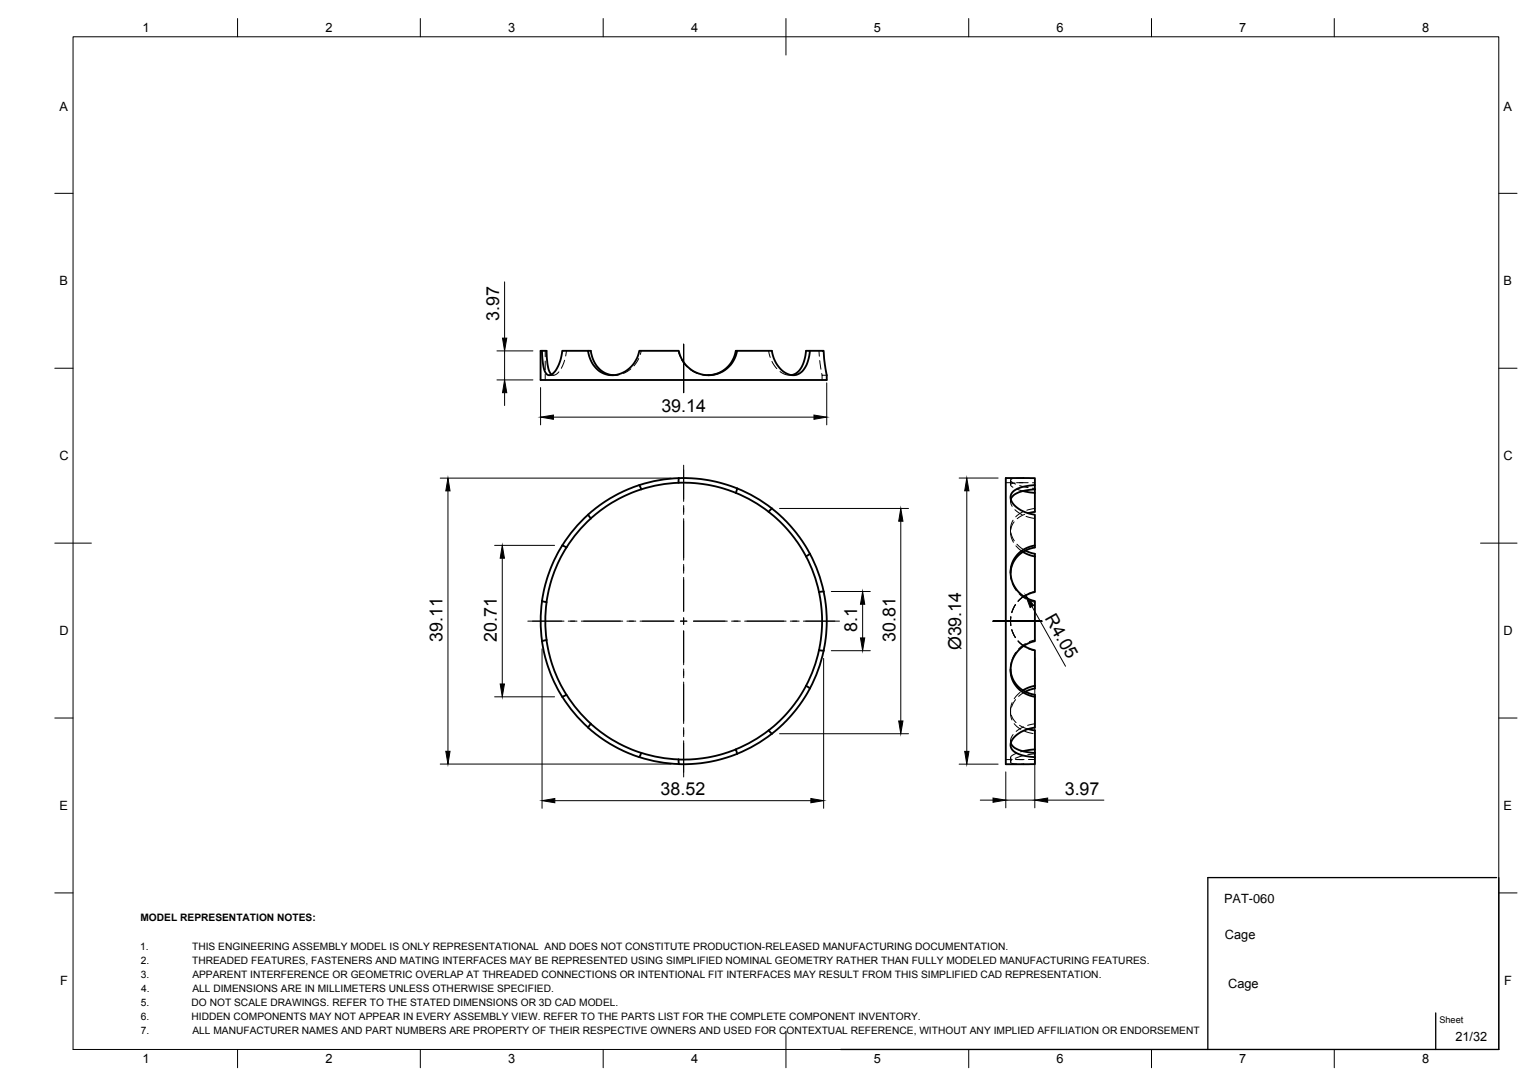
ISO-10303-21;
HEADER;
/* Generated by software containing ST-Developer
 * from STEP Tools, Inc. (www.steptools.com) 
 */

FILE_DESCRIPTION(
/* description */ ('Indexing fixture plate with plunger'),
/* implementation_level */ '2;1');

FILE_NAME(
/* name */ 'Cage.step',
/* time_stamp */ '2026-10-28T03:23:41-07:00',
/* author */ (''),
/* organization */ (''),
/* preprocessor_version */ 'ST-DEVELOPER v20.2',
/* originating_system */ 'Autodesk Translation Framework v15.17.0.0',
/* authorisation */ '');

FILE_SCHEMA (('AUTOMOTIVE_DESIGN { 1 0 10303 214 3 1 1 }'));
ENDSEC;

DATA;
#10=MECHANICAL_DESIGN_GEOMETRIC_PRESENTATION_REPRESENTATION('',(#341),#10020);
#204=SPHERICAL_SURFACE('',#5145,0.412776);
#205=SPHERICAL_SURFACE('',#5163,0.412776);
#206=SPHERICAL_SURFACE('',#5168,0.412776);
#207=SPHERICAL_SURFACE('',#5173,0.412776);
#208=SPHERICAL_SURFACE('',#5179,0.412776);
#209=SPHERICAL_SURFACE('',#5184,0.412776);
#210=SPHERICAL_SURFACE('',#5189,0.412776);
#211=SPHERICAL_SURFACE('',#5194,0.412776);
#212=SPHERICAL_SURFACE('',#5202,0.412776);
#240=B_SPLINE_CURVE_WITH_KNOTS('',3,(#8709,#8710,#8711,#8712,#8713,#8714,
#8715,#8716,#8717,#8718,#8719,#8720,#8721,#8722,#8723,#8724,#8725,#8726,
#8727,#8728,#8729,#8730),.UNSPECIFIED.,.F.,.F.,(4,2,2,2,2,2,2,2,2,2,4),
(0.0789043916784349,0.21052649634152,0.31578974451228,0.421052992683041,
0.522171766675512,0.623290540667983,0.724409314660453,0.825528088652924,
0.930791336823684,1.03605458499444,1.16767668965753),.UNSPECIFIED.);
#241=B_SPLINE_CURVE_WITH_KNOTS('',3,(#8734,#8735,#8736,#8737,#8738,#8739,
#8740,#8741,#8742,#8743,#8744,#8745,#8746,#8747,#8748,#8749,#8750,#8751,
#8752,#8753,#8754,#8755),.UNSPECIFIED.,.F.,.F.,(4,2,2,2,2,2,2,2,2,2,4),
(0.0774711646211702,0.142095081356994,0.284190162713987,0.410912155766437,
0.514012992401139,0.617113829035841,0.720214665670543,0.823315502305246,
0.950037495357694,1.09213257671469,1.15675649345051),.UNSPECIFIED.);
#242=B_SPLINE_CURVE_WITH_KNOTS('',3,(#8761,#8762,#8763,#8764,#8765,#8766,
#8767,#8768,#8769,#8770,#8771,#8772,#8773,#8774,#8775,#8776,#8777,#8778,
#8779,#8780,#8781,#8782),.UNSPECIFIED.,.F.,.F.,(4,2,2,2,2,2,2,2,2,2,4),
(0.0774711646211703,0.142095081356994,0.284190162713988,0.410912155766436,
0.514012992401139,0.617113829035841,0.720214665670544,0.823315502305246,
0.950037495357695,1.09213257671469,1.15675649345051),.UNSPECIFIED.);
#243=B_SPLINE_CURVE_WITH_KNOTS('',3,(#8786,#8787,#8788,#8789,#8790,#8791,
#8792,#8793,#8794,#8795,#8796,#8797,#8798,#8799,#8800,#8801,#8802,#8803,
#8804,#8805,#8806,#8807),.UNSPECIFIED.,.F.,.F.,(4,2,2,2,2,2,2,2,2,2,4),
(0.0774711646211702,0.142095081356994,0.284190162713988,0.410912155766436,
0.514012992401139,0.617113829035841,0.720214665670544,0.823315502305246,
0.950037495357695,1.09213257671469,1.15675649345051),.UNSPECIFIED.);
#244=B_SPLINE_CURVE_WITH_KNOTS('',3,(#8811,#8812,#8813,#8814,#8815,#8816,
#8817,#8818,#8819,#8820,#8821,#8822,#8823,#8824,#8825,#8826,#8827,#8828,
#8829,#8830,#8831,#8832),.UNSPECIFIED.,.F.,.F.,(4,2,2,2,2,2,2,2,2,2,4),
(0.0774711646211702,0.142095081356994,0.284190162713988,0.410912155766436,
0.514012992401139,0.617113829035842,0.720214665670544,0.823315502305246,
0.950037495357696,1.09213257671469,1.15675649345051),.UNSPECIFIED.);
#245=B_SPLINE_CURVE_WITH_KNOTS('',3,(#8841,#8842,#8843,#8844,#8845,#8846,
#8847,#8848,#8849,#8850,#8851,#8852,#8853,#8854,#8855,#8856,#8857,#8858,
#8859,#8860,#8861,#8862),.UNSPECIFIED.,.F.,.F.,(4,2,2,2,2,2,2,2,2,2,4),
(0.0774711646211702,0.142095081356994,0.284190162713987,0.410912155766436,
0.514012992401139,0.617113829035841,0.720214665670543,0.823315502305246,
0.950037495357695,1.09213257671469,1.15675649345051),.UNSPECIFIED.);
#246=B_SPLINE_CURVE_WITH_KNOTS('',3,(#8866,#8867,#8868,#8869,#8870,#8871,
#8872,#8873,#8874,#8875,#8876,#8877,#8878,#8879,#8880,#8881,#8882,#8883,
#8884,#8885,#8886,#8887),.UNSPECIFIED.,.F.,.F.,(4,2,2,2,2,2,2,2,2,2,4),
(0.0774711646211702,0.142095081356994,0.284190162713987,0.410912155766436,
0.514012992401139,0.617113829035841,0.720214665670543,0.823315502305246,
0.950037495357695,1.09213257671469,1.15675649345051),.UNSPECIFIED.);
#247=B_SPLINE_CURVE_WITH_KNOTS('',3,(#8891,#8892,#8893,#8894,#8895,#8896,
#8897,#8898,#8899,#8900,#8901,#8902,#8903,#8904,#8905,#8906,#8907,#8908,
#8909,#8910,#8911,#8912),.UNSPECIFIED.,.F.,.F.,(4,2,2,2,2,2,2,2,2,2,4),
(0.0774711646211703,0.142095081356994,0.284190162713988,0.410912155766437,
0.514012992401139,0.617113829035841,0.720214665670544,0.823315502305247,
0.950037495357696,1.09213257671469,1.15675649345051),.UNSPECIFIED.);
#248=B_SPLINE_CURVE_WITH_KNOTS('',3,(#8916,#8917,#8918,#8919,#8920,#8921,
#8922,#8923,#8924,#8925,#8926,#8927,#8928,#8929,#8930,#8931,#8932,#8933,
#8934,#8935,#8936,#8937),.UNSPECIFIED.,.F.,.F.,(4,2,2,2,2,2,2,2,2,2,4),
(0.0774711646211703,0.142095081356994,0.284190162713987,0.410912155766436,
0.514012992401139,0.617113829035841,0.720214665670543,0.823315502305245,
0.950037495357694,1.09213257671469,1.15675649345051),.UNSPECIFIED.);
#249=B_SPLINE_CURVE_WITH_KNOTS('',3,(#8941,#8942,#8943,#8944,#8945,#8946,
#8947,#8948,#8949,#8950,#8951,#8952,#8953,#8954,#8955,#8956,#8957,#8958,
#8959,#8960,#8961,#8962),.UNSPECIFIED.,.F.,.F.,(4,2,2,2,2,2,2,2,2,2,4),
(0.0774711646211703,0.142095081356994,0.284190162713988,0.410912155766437,
0.514012992401139,0.617113829035841,0.720214665670544,0.823315502305246,
0.950037495357695,1.09213257671469,1.15675649345051),.UNSPECIFIED.);
#250=B_SPLINE_CURVE_WITH_KNOTS('',3,(#8970,#8971,#8972,#8973,#8974,#8975,
#8976,#8977,#8978,#8979,#8980,#8981,#8982,#8983,#8984,#8985,#8986,#8987,
#8988,#8989,#8990,#8991),.UNSPECIFIED.,.F.,.F.,(4,2,2,2,2,2,2,2,2,2,4),
(0.0789043916784349,0.21052649634152,0.315789744512281,0.421052992683041,
0.522171766675512,0.623290540667983,0.724409314660453,0.825528088652924,
0.930791336823684,1.03605458499444,1.16767668965753),.UNSPECIFIED.);
#251=B_SPLINE_CURVE_WITH_KNOTS('',3,(#8999,#9000,#9001,#9002,#9003,#9004,
#9005,#9006,#9007,#9008,#9009,#9010,#9011,#9012,#9013,#9014,#9015,#9016,
#9017,#9018,#9019,#9020),.UNSPECIFIED.,.F.,.F.,(4,2,2,2,2,2,2,2,2,2,4),
(0.0789043916784348,0.210526496341521,0.315789744512281,0.421052992683042,
0.522171766675513,0.623290540667983,0.724409314660454,0.825528088652925,
0.930791336823685,1.03605458499444,1.16767668965753),.UNSPECIFIED.);
#252=B_SPLINE_CURVE_WITH_KNOTS('',3,(#9028,#9029,#9030,#9031,#9032,#9033,
#9034,#9035,#9036,#9037,#9038,#9039,#9040,#9041,#9042,#9043,#9044,#9045,
#9046,#9047,#9048,#9049),.UNSPECIFIED.,.F.,.F.,(4,2,2,2,2,2,2,2,2,2,4),
(0.0789043916784349,0.21052649634152,0.31578974451228,0.421052992683041,
0.522171766675511,0.623290540667982,0.724409314660453,0.825528088652924,
0.930791336823685,1.03605458499444,1.16767668965753),.UNSPECIFIED.);
#253=B_SPLINE_CURVE_WITH_KNOTS('',3,(#9059,#9060,#9061,#9062,#9063,#9064,
#9065,#9066,#9067,#9068,#9069,#9070,#9071,#9072,#9073,#9074,#9075,#9076,
#9077,#9078,#9079,#9080),.UNSPECIFIED.,.F.,.F.,(4,2,2,2,2,2,2,2,2,2,4),
(0.0789043916784348,0.21052649634152,0.315789744512281,0.421052992683041,
0.522171766675511,0.623290540667982,0.724409314660453,0.825528088652924,
0.930791336823684,1.03605458499444,1.16767668965753),.UNSPECIFIED.);
#254=B_SPLINE_CURVE_WITH_KNOTS('',3,(#9088,#9089,#9090,#9091,#9092,#9093,
#9094,#9095,#9096,#9097,#9098,#9099,#9100,#9101,#9102,#9103,#9104,#9105,
#9106,#9107,#9108,#9109),.UNSPECIFIED.,.F.,.F.,(4,2,2,2,2,2,2,2,2,2,4),
(0.0789043916784348,0.21052649634152,0.31578974451228,0.42105299268304,
0.522171766675511,0.623290540667982,0.724409314660453,0.825528088652924,
0.930791336823684,1.03605458499444,1.16767668965753),.UNSPECIFIED.);
#255=B_SPLINE_CURVE_WITH_KNOTS('',3,(#9117,#9118,#9119,#9120,#9121,#9122,
#9123,#9124,#9125,#9126,#9127,#9128,#9129,#9130,#9131,#9132,#9133,#9134,
#9135,#9136,#9137,#9138),.UNSPECIFIED.,.F.,.F.,(4,2,2,2,2,2,2,2,2,2,4),
(0.0789043916784348,0.21052649634152,0.315789744512281,0.421052992683041,
0.522171766675512,0.623290540667982,0.724409314660453,0.825528088652924,
0.930791336823684,1.03605458499444,1.16767668965753),.UNSPECIFIED.);
#256=B_SPLINE_CURVE_WITH_KNOTS('',3,(#9146,#9147,#9148,#9149,#9150,#9151,
#9152,#9153,#9154,#9155,#9156,#9157,#9158,#9159,#9160,#9161,#9162,#9163,
#9164,#9165,#9166,#9167),.UNSPECIFIED.,.F.,.F.,(4,2,2,2,2,2,2,2,2,2,4),
(0.0789043916784349,0.21052649634152,0.31578974451228,0.42105299268304,
0.522171766675511,0.623290540667982,0.724409314660453,0.825528088652924,
0.930791336823684,1.03605458499444,1.16767668965753),.UNSPECIFIED.);
#257=B_SPLINE_CURVE_WITH_KNOTS('',3,(#9176,#9177,#9178,#9179,#9180,#9181,
#9182,#9183,#9184,#9185,#9186,#9187,#9188,#9189,#9190,#9191,#9192,#9193,
#9194,#9195,#9196,#9197),.UNSPECIFIED.,.F.,.F.,(4,2,2,2,2,2,2,2,2,2,4),
(0.0789043916784348,0.21052649634152,0.31578974451228,0.42105299268304,
0.522171766675511,0.623290540667982,0.724409314660453,0.825528088652924,
0.930791336823684,1.03605458499444,1.16767668965753),.UNSPECIFIED.);
#279=SHAPE_REPRESENTATION_RELATIONSHIP('SRR','None',#10154,#306);
#306=ADVANCED_BREP_SHAPE_REPRESENTATION('',(#376),#10007);
#341=STYLED_ITEM('',(#10368),#376);
#376=MANIFOLD_SOLID_BREP('Continuous crown cage',#4596);
#435=FACE_BOUND('',#1135,.T.);
#587=PLANE('',#5160);
#588=PLANE('',#5165);
#589=PLANE('',#5170);
#590=PLANE('',#5175);
#591=PLANE('',#5181);
#592=PLANE('',#5186);
#593=PLANE('',#5191);
#594=PLANE('',#5200);
#595=PLANE('',#5204);
#596=PLANE('',#5205);
#781=FACE_OUTER_BOUND('',#1115,.T.);
#782=FACE_OUTER_BOUND('',#1116,.T.);
#783=FACE_OUTER_BOUND('',#1117,.T.);
#784=FACE_OUTER_BOUND('',#1118,.T.);
#785=FACE_OUTER_BOUND('',#1119,.T.);
#786=FACE_OUTER_BOUND('',#1120,.T.);
#787=FACE_OUTER_BOUND('',#1121,.T.);
#788=FACE_OUTER_BOUND('',#1122,.T.);
#789=FACE_OUTER_BOUND('',#1123,.T.);
#790=FACE_OUTER_BOUND('',#1124,.T.);
#791=FACE_OUTER_BOUND('',#1125,.T.);
#792=FACE_OUTER_BOUND('',#1126,.T.);
#793=FACE_OUTER_BOUND('',#1127,.T.);
#794=FACE_OUTER_BOUND('',#1128,.T.);
#795=FACE_OUTER_BOUND('',#1129,.T.);
#796=FACE_OUTER_BOUND('',#1130,.T.);
#797=FACE_OUTER_BOUND('',#1131,.T.);
#798=FACE_OUTER_BOUND('',#1132,.T.);
#799=FACE_OUTER_BOUND('',#1133,.T.);
#800=FACE_OUTER_BOUND('',#1134,.T.);
#801=FACE_OUTER_BOUND('',#1136,.T.);
#1115=EDGE_LOOP('',(#3453,#3454,#3455,#3456));
#1116=EDGE_LOOP('',(#3457,#3458,#3459,#3460,#3461,#3462,#3463,#3464,#3465,
#3466,#3467,#3468,#3469,#3470,#3471,#3472,#3473,#3474,#3475,#3476,#3477,
#3478));
#1117=EDGE_LOOP('',(#3479,#3480,#3481,#3482));
#1118=EDGE_LOOP('',(#3483,#3484,#3485,#3486));
#1119=EDGE_LOOP('',(#3487,#3488,#3489,#3490));
#1120=EDGE_LOOP('',(#3491,#3492,#3493,#3494));
#1121=EDGE_LOOP('',(#3495,#3496,#3497,#3498));
#1122=EDGE_LOOP('',(#3499,#3500,#3501,#3502));
#1123=EDGE_LOOP('',(#3503,#3504,#3505,#3506,#3507,#3508));
#1124=EDGE_LOOP('',(#3509,#3510,#3511,#3512));
#1125=EDGE_LOOP('',(#3513,#3514,#3515,#3516));
#1126=EDGE_LOOP('',(#3517,#3518,#3519,#3520));
#1127=EDGE_LOOP('',(#3521,#3522,#3523,#3524));
#1128=EDGE_LOOP('',(#3525,#3526,#3527,#3528));
#1129=EDGE_LOOP('',(#3529,#3530,#3531,#3532));
#1130=EDGE_LOOP('',(#3533,#3534,#3535,#3536));
#1131=EDGE_LOOP('',(#3537,#3538,#3539,#3540,#3541,#3542,#3543,#3544,#3545,
#3546,#3547,#3548,#3549,#3550,#3551,#3552,#3553,#3554,#3555,#3556,#3557,
#3558));
#1132=EDGE_LOOP('',(#3559,#3560,#3561,#3562));
#1133=EDGE_LOOP('',(#3563,#3564,#3565,#3566));
#1134=EDGE_LOOP('',(#3567));
#1135=EDGE_LOOP('',(#3568));
#1136=EDGE_LOOP('',(#3569,#3570,#3571,#3572));
#1473=LINE('',#8836,#1693);
#1474=LINE('',#9172,#1694);
#1693=VECTOR('',#6146,1.956752);
#1694=VECTOR('',#6237,1.893248);
#1940=CIRCLE('',#5146,0.405071403305639);
#1941=CIRCLE('',#5147,0.405071403305639);
#1942=CIRCLE('',#5149,1.956752);
#1943=CIRCLE('',#5150,1.956752);
#1944=CIRCLE('',#5151,1.956752);
#1945=CIRCLE('',#5152,1.956752);
#1946=CIRCLE('',#5153,1.956752);
#1947=CIRCLE('',#5154,1.956752);
#1948=CIRCLE('',#5155,1.956752);
#1949=CIRCLE('',#5156,1.956752);
#1950=CIRCLE('',#5157,1.956752);
#1951=CIRCLE('',#5158,1.956752);
#1952=CIRCLE('',#5159,1.956752);
#1953=CIRCLE('',#5161,1.893248);
#1954=CIRCLE('',#5162,0.405071403305639);
#1955=CIRCLE('',#5164,0.405071403305639);
#1956=CIRCLE('',#5166,1.893248);
#1957=CIRCLE('',#5167,0.405071403305639);
#1958=CIRCLE('',#5169,0.405071403305639);
#1959=CIRCLE('',#5171,1.893248);
#1960=CIRCLE('',#5172,0.405071403305639);
#1961=CIRCLE('',#5174,0.405071403305639);
#1962=CIRCLE('',#5176,1.893248);
#1963=CIRCLE('',#5177,1.893248);
#1964=CIRCLE('',#5178,0.405071403305639);
#1965=CIRCLE('',#5180,0.405071403305639);
#1966=CIRCLE('',#5182,1.893248);
#1967=CIRCLE('',#5183,0.405071403305639);
#1968=CIRCLE('',#5185,0.405071403305639);
#1969=CIRCLE('',#5187,1.893248);
#1970=CIRCLE('',#5188,0.405071403305639);
#1971=CIRCLE('',#5190,0.405071403305639);
#1972=CIRCLE('',#5192,1.893248);
#1973=CIRCLE('',#5193,0.405071403305639);
#1974=CIRCLE('',#5195,0.405071403305639);
#1975=CIRCLE('',#5197,1.893248);
#1976=CIRCLE('',#5198,1.893248);
#1977=CIRCLE('',#5199,1.893248);
#1978=CIRCLE('',#5201,0.405071403305639);
#1979=CIRCLE('',#5203,0.405071403305639);
#2275=VERTEX_POINT('',#8707);
#2276=VERTEX_POINT('',#8708);
#2277=VERTEX_POINT('',#8731);
#2278=VERTEX_POINT('',#8733);
#2279=VERTEX_POINT('',#8758);
#2280=VERTEX_POINT('',#8760);
#2281=VERTEX_POINT('',#8783);
#2282=VERTEX_POINT('',#8785);
#2283=VERTEX_POINT('',#8808);
#2284=VERTEX_POINT('',#8810);
#2285=VERTEX_POINT('',#8833);
#2286=VERTEX_POINT('',#8835);
#2287=VERTEX_POINT('',#8838);
#2288=VERTEX_POINT('',#8840);
#2289=VERTEX_POINT('',#8863);
#2290=VERTEX_POINT('',#8865);
#2291=VERTEX_POINT('',#8888);
#2292=VERTEX_POINT('',#8890);
#2293=VERTEX_POINT('',#8913);
#2294=VERTEX_POINT('',#8915);
#2295=VERTEX_POINT('',#8938);
#2296=VERTEX_POINT('',#8940);
#2297=VERTEX_POINT('',#8965);
#2298=VERTEX_POINT('',#8969);
#2299=VERTEX_POINT('',#8994);
#2300=VERTEX_POINT('',#8998);
#2301=VERTEX_POINT('',#9023);
#2302=VERTEX_POINT('',#9027);
#2303=VERTEX_POINT('',#9052);
#2304=VERTEX_POINT('',#9054);
#2305=VERTEX_POINT('',#9058);
#2306=VERTEX_POINT('',#9083);
#2307=VERTEX_POINT('',#9087);
#2308=VERTEX_POINT('',#9112);
#2309=VERTEX_POINT('',#9116);
#2310=VERTEX_POINT('',#9141);
#2311=VERTEX_POINT('',#9145);
#2312=VERTEX_POINT('',#9170);
#2313=VERTEX_POINT('',#9173);
#2314=VERTEX_POINT('',#9175);
#2706=EDGE_CURVE('',#2275,#2276,#240,.T.);
#2707=EDGE_CURVE('',#2277,#2275,#1940,.T.);
#2708=EDGE_CURVE('',#2278,#2277,#241,.T.);
#2709=EDGE_CURVE('',#2276,#2278,#1941,.T.);
#2710=EDGE_CURVE('',#2279,#2277,#1942,.T.);
#2711=EDGE_CURVE('',#2279,#2280,#242,.T.);
#2712=EDGE_CURVE('',#2281,#2280,#1943,.T.);
#2713=EDGE_CURVE('',#2281,#2282,#243,.T.);
#2714=EDGE_CURVE('',#2283,#2282,#1944,.T.);
#2715=EDGE_CURVE('',#2283,#2284,#244,.T.);
#2716=EDGE_CURVE('',#2285,#2284,#1945,.T.);
#2717=EDGE_CURVE('',#2285,#2286,#1473,.T.);
#2718=EDGE_CURVE('',#2286,#2286,#1946,.T.);
#2719=EDGE_CURVE('',#2287,#2285,#1947,.T.);
#2720=EDGE_CURVE('',#2287,#2288,#245,.T.);
#2721=EDGE_CURVE('',#2289,#2288,#1948,.T.);
#2722=EDGE_CURVE('',#2289,#2290,#246,.T.);
#2723=EDGE_CURVE('',#2291,#2290,#1949,.T.);
#2724=EDGE_CURVE('',#2291,#2292,#247,.T.);
#2725=EDGE_CURVE('',#2293,#2292,#1950,.T.);
#2726=EDGE_CURVE('',#2293,#2294,#248,.T.);
#2727=EDGE_CURVE('',#2295,#2294,#1951,.T.);
#2728=EDGE_CURVE('',#2295,#2296,#249,.T.);
#2729=EDGE_CURVE('',#2278,#2296,#1952,.T.);
#2730=EDGE_CURVE('',#2275,#2297,#1953,.T.);
#2731=EDGE_CURVE('',#2297,#2279,#1954,.T.);
#2732=EDGE_CURVE('',#2298,#2297,#250,.T.);
#2733=EDGE_CURVE('',#2280,#2298,#1955,.T.);
#2734=EDGE_CURVE('',#2298,#2299,#1956,.T.);
#2735=EDGE_CURVE('',#2299,#2281,#1957,.T.);
#2736=EDGE_CURVE('',#2300,#2299,#251,.T.);
#2737=EDGE_CURVE('',#2282,#2300,#1958,.T.);
#2738=EDGE_CURVE('',#2300,#2301,#1959,.T.);
#2739=EDGE_CURVE('',#2301,#2283,#1960,.T.);
#2740=EDGE_CURVE('',#2302,#2301,#252,.T.);
#2741=EDGE_CURVE('',#2284,#2302,#1961,.T.);
#2742=EDGE_CURVE('',#2302,#2303,#1962,.T.);
#2743=EDGE_CURVE('',#2303,#2304,#1963,.T.);
#2744=EDGE_CURVE('',#2304,#2287,#1964,.T.);
#2745=EDGE_CURVE('',#2305,#2304,#253,.T.);
#2746=EDGE_CURVE('',#2288,#2305,#1965,.T.);
#2747=EDGE_CURVE('',#2305,#2306,#1966,.T.);
#2748=EDGE_CURVE('',#2306,#2289,#1967,.T.);
#2749=EDGE_CURVE('',#2307,#2306,#254,.T.);
#2750=EDGE_CURVE('',#2290,#2307,#1968,.T.);
#2751=EDGE_CURVE('',#2307,#2308,#1969,.T.);
#2752=EDGE_CURVE('',#2308,#2291,#1970,.T.);
#2753=EDGE_CURVE('',#2309,#2308,#255,.T.);
#2754=EDGE_CURVE('',#2292,#2309,#1971,.T.);
#2755=EDGE_CURVE('',#2309,#2310,#1972,.T.);
#2756=EDGE_CURVE('',#2310,#2293,#1973,.T.);
#2757=EDGE_CURVE('',#2311,#2310,#256,.T.);
#2758=EDGE_CURVE('',#2294,#2311,#1974,.T.);
#2759=EDGE_CURVE('',#2312,#2312,#1975,.T.);
#2760=EDGE_CURVE('',#2312,#2303,#1474,.T.);
#2761=EDGE_CURVE('',#2313,#2276,#1976,.T.);
#2762=EDGE_CURVE('',#2313,#2314,#257,.T.);
#2763=EDGE_CURVE('',#2311,#2314,#1977,.T.);
#2764=EDGE_CURVE('',#2296,#2313,#1978,.T.);
#2765=EDGE_CURVE('',#2314,#2295,#1979,.T.);
#3453=ORIENTED_EDGE('',*,*,#2706,.F.);
#3454=ORIENTED_EDGE('',*,*,#2707,.F.);
#3455=ORIENTED_EDGE('',*,*,#2708,.F.);
#3456=ORIENTED_EDGE('',*,*,#2709,.F.);
#3457=ORIENTED_EDGE('',*,*,#2708,.T.);
#3458=ORIENTED_EDGE('',*,*,#2710,.F.);
#3459=ORIENTED_EDGE('',*,*,#2711,.T.);
#3460=ORIENTED_EDGE('',*,*,#2712,.F.);
#3461=ORIENTED_EDGE('',*,*,#2713,.T.);
#3462=ORIENTED_EDGE('',*,*,#2714,.F.);
#3463=ORIENTED_EDGE('',*,*,#2715,.T.);
#3464=ORIENTED_EDGE('',*,*,#2716,.F.);
#3465=ORIENTED_EDGE('',*,*,#2717,.T.);
#3466=ORIENTED_EDGE('',*,*,#2718,.F.);
#3467=ORIENTED_EDGE('',*,*,#2717,.F.);
#3468=ORIENTED_EDGE('',*,*,#2719,.F.);
#3469=ORIENTED_EDGE('',*,*,#2720,.T.);
#3470=ORIENTED_EDGE('',*,*,#2721,.F.);
#3471=ORIENTED_EDGE('',*,*,#2722,.T.);
#3472=ORIENTED_EDGE('',*,*,#2723,.F.);
#3473=ORIENTED_EDGE('',*,*,#2724,.T.);
#3474=ORIENTED_EDGE('',*,*,#2725,.F.);
#3475=ORIENTED_EDGE('',*,*,#2726,.T.);
#3476=ORIENTED_EDGE('',*,*,#2727,.F.);
#3477=ORIENTED_EDGE('',*,*,#2728,.T.);
#3478=ORIENTED_EDGE('',*,*,#2729,.F.);
#3479=ORIENTED_EDGE('',*,*,#2707,.T.);
#3480=ORIENTED_EDGE('',*,*,#2730,.T.);
#3481=ORIENTED_EDGE('',*,*,#2731,.T.);
#3482=ORIENTED_EDGE('',*,*,#2710,.T.);
#3483=ORIENTED_EDGE('',*,*,#2732,.F.);
#3484=ORIENTED_EDGE('',*,*,#2733,.F.);
#3485=ORIENTED_EDGE('',*,*,#2711,.F.);
#3486=ORIENTED_EDGE('',*,*,#2731,.F.);
#3487=ORIENTED_EDGE('',*,*,#2733,.T.);
#3488=ORIENTED_EDGE('',*,*,#2734,.T.);
#3489=ORIENTED_EDGE('',*,*,#2735,.T.);
#3490=ORIENTED_EDGE('',*,*,#2712,.T.);
#3491=ORIENTED_EDGE('',*,*,#2736,.F.);
#3492=ORIENTED_EDGE('',*,*,#2737,.F.);
#3493=ORIENTED_EDGE('',*,*,#2713,.F.);
#3494=ORIENTED_EDGE('',*,*,#2735,.F.);
#3495=ORIENTED_EDGE('',*,*,#2737,.T.);
#3496=ORIENTED_EDGE('',*,*,#2738,.T.);
#3497=ORIENTED_EDGE('',*,*,#2739,.T.);
#3498=ORIENTED_EDGE('',*,*,#2714,.T.);
#3499=ORIENTED_EDGE('',*,*,#2740,.F.);
#3500=ORIENTED_EDGE('',*,*,#2741,.F.);
#3501=ORIENTED_EDGE('',*,*,#2715,.F.);
#3502=ORIENTED_EDGE('',*,*,#2739,.F.);
#3503=ORIENTED_EDGE('',*,*,#2741,.T.);
#3504=ORIENTED_EDGE('',*,*,#2742,.T.);
#3505=ORIENTED_EDGE('',*,*,#2743,.T.);
#3506=ORIENTED_EDGE('',*,*,#2744,.T.);
#3507=ORIENTED_EDGE('',*,*,#2719,.T.);
#3508=ORIENTED_EDGE('',*,*,#2716,.T.);
#3509=ORIENTED_EDGE('',*,*,#2745,.F.);
#3510=ORIENTED_EDGE('',*,*,#2746,.F.);
#3511=ORIENTED_EDGE('',*,*,#2720,.F.);
#3512=ORIENTED_EDGE('',*,*,#2744,.F.);
#3513=ORIENTED_EDGE('',*,*,#2746,.T.);
#3514=ORIENTED_EDGE('',*,*,#2747,.T.);
#3515=ORIENTED_EDGE('',*,*,#2748,.T.);
#3516=ORIENTED_EDGE('',*,*,#2721,.T.);
#3517=ORIENTED_EDGE('',*,*,#2749,.F.);
#3518=ORIENTED_EDGE('',*,*,#2750,.F.);
#3519=ORIENTED_EDGE('',*,*,#2722,.F.);
#3520=ORIENTED_EDGE('',*,*,#2748,.F.);
#3521=ORIENTED_EDGE('',*,*,#2750,.T.);
#3522=ORIENTED_EDGE('',*,*,#2751,.T.);
#3523=ORIENTED_EDGE('',*,*,#2752,.T.);
#3524=ORIENTED_EDGE('',*,*,#2723,.T.);
#3525=ORIENTED_EDGE('',*,*,#2753,.F.);
#3526=ORIENTED_EDGE('',*,*,#2754,.F.);
#3527=ORIENTED_EDGE('',*,*,#2724,.F.);
#3528=ORIENTED_EDGE('',*,*,#2752,.F.);
#3529=ORIENTED_EDGE('',*,*,#2754,.T.);
#3530=ORIENTED_EDGE('',*,*,#2755,.T.);
#3531=ORIENTED_EDGE('',*,*,#2756,.T.);
#3532=ORIENTED_EDGE('',*,*,#2725,.T.);
#3533=ORIENTED_EDGE('',*,*,#2726,.F.);
#3534=ORIENTED_EDGE('',*,*,#2756,.F.);
#3535=ORIENTED_EDGE('',*,*,#2757,.F.);
#3536=ORIENTED_EDGE('',*,*,#2758,.F.);
#3537=ORIENTED_EDGE('',*,*,#2759,.F.);
#3538=ORIENTED_EDGE('',*,*,#2760,.T.);
#3539=ORIENTED_EDGE('',*,*,#2742,.F.);
#3540=ORIENTED_EDGE('',*,*,#2740,.T.);
#3541=ORIENTED_EDGE('',*,*,#2738,.F.);
#3542=ORIENTED_EDGE('',*,*,#2736,.T.);
#3543=ORIENTED_EDGE('',*,*,#2734,.F.);
#3544=ORIENTED_EDGE('',*,*,#2732,.T.);
#3545=ORIENTED_EDGE('',*,*,#2730,.F.);
#3546=ORIENTED_EDGE('',*,*,#2706,.T.);
#3547=ORIENTED_EDGE('',*,*,#2761,.F.);
#3548=ORIENTED_EDGE('',*,*,#2762,.T.);
#3549=ORIENTED_EDGE('',*,*,#2763,.F.);
#3550=ORIENTED_EDGE('',*,*,#2757,.T.);
#3551=ORIENTED_EDGE('',*,*,#2755,.F.);
#3552=ORIENTED_EDGE('',*,*,#2753,.T.);
#3553=ORIENTED_EDGE('',*,*,#2751,.F.);
#3554=ORIENTED_EDGE('',*,*,#2749,.T.);
#3555=ORIENTED_EDGE('',*,*,#2747,.F.);
#3556=ORIENTED_EDGE('',*,*,#2745,.T.);
#3557=ORIENTED_EDGE('',*,*,#2743,.F.);
#3558=ORIENTED_EDGE('',*,*,#2760,.F.);
#3559=ORIENTED_EDGE('',*,*,#2709,.T.);
#3560=ORIENTED_EDGE('',*,*,#2729,.T.);
#3561=ORIENTED_EDGE('',*,*,#2764,.T.);
#3562=ORIENTED_EDGE('',*,*,#2761,.T.);
#3563=ORIENTED_EDGE('',*,*,#2728,.F.);
#3564=ORIENTED_EDGE('',*,*,#2765,.F.);
#3565=ORIENTED_EDGE('',*,*,#2762,.F.);
#3566=ORIENTED_EDGE('',*,*,#2764,.F.);
#3567=ORIENTED_EDGE('',*,*,#2718,.T.);
#3568=ORIENTED_EDGE('',*,*,#2759,.T.);
#3569=ORIENTED_EDGE('',*,*,#2758,.T.);
#3570=ORIENTED_EDGE('',*,*,#2763,.T.);
#3571=ORIENTED_EDGE('',*,*,#2765,.T.);
#3572=ORIENTED_EDGE('',*,*,#2727,.T.);
#4209=CYLINDRICAL_SURFACE('',#5148,1.956752);
#4210=CYLINDRICAL_SURFACE('',#5196,1.893248);
#4396=ADVANCED_FACE('',(#781),#204,.F.);
#4397=ADVANCED_FACE('',(#782),#4209,.T.);
#4398=ADVANCED_FACE('',(#783),#587,.T.);
#4399=ADVANCED_FACE('',(#784),#205,.F.);
#4400=ADVANCED_FACE('',(#785),#588,.T.);
#4401=ADVANCED_FACE('',(#786),#206,.F.);
#4402=ADVANCED_FACE('',(#787),#589,.T.);
#4403=ADVANCED_FACE('',(#788),#207,.F.);
#4404=ADVANCED_FACE('',(#789),#590,.T.);
#4405=ADVANCED_FACE('',(#790),#208,.F.);
#4406=ADVANCED_FACE('',(#791),#591,.T.);
#4407=ADVANCED_FACE('',(#792),#209,.F.);
#4408=ADVANCED_FACE('',(#793),#592,.T.);
#4409=ADVANCED_FACE('',(#794),#210,.F.);
#4410=ADVANCED_FACE('',(#795),#593,.T.);
#4411=ADVANCED_FACE('',(#796),#211,.F.);
#4412=ADVANCED_FACE('',(#797),#4210,.F.);
#4413=ADVANCED_FACE('',(#798),#594,.T.);
#4414=ADVANCED_FACE('',(#799),#212,.F.);
#4415=ADVANCED_FACE('',(#800,#435),#595,.T.);
#4416=ADVANCED_FACE('',(#801),#596,.T.);
#4596=CLOSED_SHELL('',(#4396,#4397,#4398,#4399,#4400,#4401,#4402,#4403,
#4404,#4405,#4406,#4407,#4408,#4409,#4410,#4411,#4412,#4413,#4414,#4415,
#4416));
#5144=AXIS2_PLACEMENT_3D('',#8705,#6128,#6129);
#5145=AXIS2_PLACEMENT_3D('',#8706,#6130,#6131);
#5146=AXIS2_PLACEMENT_3D('',#8732,#6132,#6133);
#5147=AXIS2_PLACEMENT_3D('',#8756,#6134,#6135);
#5148=AXIS2_PLACEMENT_3D('',#8757,#6136,#6137);
#5149=AXIS2_PLACEMENT_3D('',#8759,#6138,#6139);
#5150=AXIS2_PLACEMENT_3D('',#8784,#6140,#6141);
#5151=AXIS2_PLACEMENT_3D('',#8809,#6142,#6143);
#5152=AXIS2_PLACEMENT_3D('',#8834,#6144,#6145);
#5153=AXIS2_PLACEMENT_3D('',#8837,#6147,#6148);
#5154=AXIS2_PLACEMENT_3D('',#8839,#6149,#6150);
#5155=AXIS2_PLACEMENT_3D('',#8864,#6151,#6152);
#5156=AXIS2_PLACEMENT_3D('',#8889,#6153,#6154);
#5157=AXIS2_PLACEMENT_3D('',#8914,#6155,#6156);
#5158=AXIS2_PLACEMENT_3D('',#8939,#6157,#6158);
#5159=AXIS2_PLACEMENT_3D('',#8963,#6159,#6160);
#5160=AXIS2_PLACEMENT_3D('',#8964,#6161,#6162);
#5161=AXIS2_PLACEMENT_3D('',#8966,#6163,#6164);
#5162=AXIS2_PLACEMENT_3D('',#8967,#6165,#6166);
#5163=AXIS2_PLACEMENT_3D('',#8968,#6167,#6168);
#5164=AXIS2_PLACEMENT_3D('',#8992,#6169,#6170);
#5165=AXIS2_PLACEMENT_3D('',#8993,#6171,#6172);
#5166=AXIS2_PLACEMENT_3D('',#8995,#6173,#6174);
#5167=AXIS2_PLACEMENT_3D('',#8996,#6175,#6176);
#5168=AXIS2_PLACEMENT_3D('',#8997,#6177,#6178);
#5169=AXIS2_PLACEMENT_3D('',#9021,#6179,#6180);
#5170=AXIS2_PLACEMENT_3D('',#9022,#6181,#6182);
#5171=AXIS2_PLACEMENT_3D('',#9024,#6183,#6184);
#5172=AXIS2_PLACEMENT_3D('',#9025,#6185,#6186);
#5173=AXIS2_PLACEMENT_3D('',#9026,#6187,#6188);
#5174=AXIS2_PLACEMENT_3D('',#9050,#6189,#6190);
#5175=AXIS2_PLACEMENT_3D('',#9051,#6191,#6192);
#5176=AXIS2_PLACEMENT_3D('',#9053,#6193,#6194);
#5177=AXIS2_PLACEMENT_3D('',#9055,#6195,#6196);
#5178=AXIS2_PLACEMENT_3D('',#9056,#6197,#6198);
#5179=AXIS2_PLACEMENT_3D('',#9057,#6199,#6200);
#5180=AXIS2_PLACEMENT_3D('',#9081,#6201,#6202);
#5181=AXIS2_PLACEMENT_3D('',#9082,#6203,#6204);
#5182=AXIS2_PLACEMENT_3D('',#9084,#6205,#6206);
#5183=AXIS2_PLACEMENT_3D('',#9085,#6207,#6208);
#5184=AXIS2_PLACEMENT_3D('',#9086,#6209,#6210);
#5185=AXIS2_PLACEMENT_3D('',#9110,#6211,#6212);
#5186=AXIS2_PLACEMENT_3D('',#9111,#6213,#6214);
#5187=AXIS2_PLACEMENT_3D('',#9113,#6215,#6216);
#5188=AXIS2_PLACEMENT_3D('',#9114,#6217,#6218);
#5189=AXIS2_PLACEMENT_3D('',#9115,#6219,#6220);
#5190=AXIS2_PLACEMENT_3D('',#9139,#6221,#6222);
#5191=AXIS2_PLACEMENT_3D('',#9140,#6223,#6224);
#5192=AXIS2_PLACEMENT_3D('',#9142,#6225,#6226);
#5193=AXIS2_PLACEMENT_3D('',#9143,#6227,#6228);
#5194=AXIS2_PLACEMENT_3D('',#9144,#6229,#6230);
#5195=AXIS2_PLACEMENT_3D('',#9168,#6231,#6232);
#5196=AXIS2_PLACEMENT_3D('',#9169,#6233,#6234);
#5197=AXIS2_PLACEMENT_3D('',#9171,#6235,#6236);
#5198=AXIS2_PLACEMENT_3D('',#9174,#6238,#6239);
#5199=AXIS2_PLACEMENT_3D('',#9198,#6240,#6241);
#5200=AXIS2_PLACEMENT_3D('',#9199,#6242,#6243);
#5201=AXIS2_PLACEMENT_3D('',#9200,#6244,#6245);
#5202=AXIS2_PLACEMENT_3D('',#9201,#6246,#6247);
#5203=AXIS2_PLACEMENT_3D('',#9202,#6248,#6249);
#5204=AXIS2_PLACEMENT_3D('',#9203,#6250,#6251);
#5205=AXIS2_PLACEMENT_3D('',#9204,#6252,#6253);
#6128=DIRECTION('axis',(0.,0.,1.));
#6129=DIRECTION('refdir',(1.,0.,0.));
#6130=DIRECTION('center_axis',(0.,0.,1.));
#6131=DIRECTION('ref_axis',(1.,0.,0.));
#6132=DIRECTION('center_axis',(0.,-1.,0.));
#6133=DIRECTION('ref_axis',(0.,0.,-1.));
#6134=DIRECTION('center_axis',(0.,-1.,0.));
#6135=DIRECTION('ref_axis',(0.,0.,-1.));
#6136=DIRECTION('center_axis',(0.,1.,0.));
#6137=DIRECTION('ref_axis',(1.,0.,0.));
#6138=DIRECTION('center_axis',(0.,1.,0.));
#6139=DIRECTION('ref_axis',(1.,0.,0.));
#6140=DIRECTION('center_axis',(0.,1.,0.));
#6141=DIRECTION('ref_axis',(1.,0.,0.));
#6142=DIRECTION('center_axis',(0.,1.,0.));
#6143=DIRECTION('ref_axis',(1.,0.,0.));
#6144=DIRECTION('center_axis',(0.,1.,0.));
#6145=DIRECTION('ref_axis',(1.,0.,0.));
#6146=DIRECTION('',(0.,-1.,0.));
#6147=DIRECTION('center_axis',(0.,-1.,0.));
#6148=DIRECTION('ref_axis',(1.,0.,0.));
#6149=DIRECTION('center_axis',(0.,1.,0.));
#6150=DIRECTION('ref_axis',(1.,0.,0.));
#6151=DIRECTION('center_axis',(0.,1.,0.));
#6152=DIRECTION('ref_axis',(1.,0.,0.));
#6153=DIRECTION('center_axis',(0.,1.,0.));
#6154=DIRECTION('ref_axis',(1.,0.,0.));
#6155=DIRECTION('center_axis',(0.,1.,0.));
#6156=DIRECTION('ref_axis',(1.,0.,0.));
#6157=DIRECTION('center_axis',(0.,1.,0.));
#6158=DIRECTION('ref_axis',(1.,0.,0.));
#6159=DIRECTION('center_axis',(0.,1.,0.));
#6160=DIRECTION('ref_axis',(1.,0.,0.));
#6161=DIRECTION('center_axis',(0.,1.,0.));
#6162=DIRECTION('ref_axis',(1.,0.,0.));
#6163=DIRECTION('center_axis',(0.,-1.,0.));
#6164=DIRECTION('ref_axis',(1.,0.,0.));
#6165=DIRECTION('center_axis',(0.,-1.,0.));
#6166=DIRECTION('ref_axis',(0.,0.,-1.));
#6167=DIRECTION('center_axis',(0.,0.,1.));
#6168=DIRECTION('ref_axis',(1.,0.,0.));
#6169=DIRECTION('center_axis',(0.,-1.,0.));
#6170=DIRECTION('ref_axis',(0.,0.,-1.));
#6171=DIRECTION('center_axis',(0.,1.,0.));
#6172=DIRECTION('ref_axis',(1.,0.,0.));
#6173=DIRECTION('center_axis',(0.,-1.,0.));
#6174=DIRECTION('ref_axis',(1.,0.,0.));
#6175=DIRECTION('center_axis',(0.,-1.,0.));
#6176=DIRECTION('ref_axis',(0.,0.,-1.));
#6177=DIRECTION('center_axis',(0.,0.,1.));
#6178=DIRECTION('ref_axis',(1.,0.,0.));
#6179=DIRECTION('center_axis',(0.,-1.,0.));
#6180=DIRECTION('ref_axis',(0.,0.,-1.));
#6181=DIRECTION('center_axis',(0.,1.,0.));
#6182=DIRECTION('ref_axis',(1.,0.,0.));
#6183=DIRECTION('center_axis',(0.,-1.,0.));
#6184=DIRECTION('ref_axis',(1.,0.,0.));
#6185=DIRECTION('center_axis',(0.,-1.,0.));
#6186=DIRECTION('ref_axis',(0.,0.,-1.));
#6187=DIRECTION('center_axis',(0.,0.,1.));
#6188=DIRECTION('ref_axis',(1.,0.,0.));
#6189=DIRECTION('center_axis',(0.,-1.,0.));
#6190=DIRECTION('ref_axis',(0.,0.,-1.));
#6191=DIRECTION('center_axis',(0.,1.,0.));
#6192=DIRECTION('ref_axis',(1.,0.,0.));
#6193=DIRECTION('center_axis',(0.,-1.,0.));
#6194=DIRECTION('ref_axis',(1.,0.,0.));
#6195=DIRECTION('center_axis',(0.,-1.,0.));
#6196=DIRECTION('ref_axis',(1.,0.,0.));
#6197=DIRECTION('center_axis',(0.,-1.,0.));
#6198=DIRECTION('ref_axis',(0.,0.,-1.));
#6199=DIRECTION('center_axis',(0.,0.,1.));
#6200=DIRECTION('ref_axis',(1.,0.,0.));
#6201=DIRECTION('center_axis',(0.,-1.,0.));
#6202=DIRECTION('ref_axis',(0.,0.,-1.));
#6203=DIRECTION('center_axis',(0.,1.,0.));
#6204=DIRECTION('ref_axis',(1.,0.,0.));
#6205=DIRECTION('center_axis',(0.,-1.,0.));
#6206=DIRECTION('ref_axis',(1.,0.,0.));
#6207=DIRECTION('center_axis',(0.,-1.,0.));
#6208=DIRECTION('ref_axis',(0.,0.,-1.));
#6209=DIRECTION('center_axis',(0.,0.,1.));
#6210=DIRECTION('ref_axis',(1.,0.,0.));
#6211=DIRECTION('center_axis',(0.,-1.,0.));
#6212=DIRECTION('ref_axis',(0.,0.,-1.));
#6213=DIRECTION('center_axis',(0.,1.,0.));
#6214=DIRECTION('ref_axis',(1.,0.,0.));
#6215=DIRECTION('center_axis',(0.,-1.,0.));
#6216=DIRECTION('ref_axis',(1.,0.,0.));
#6217=DIRECTION('center_axis',(0.,-1.,0.));
#6218=DIRECTION('ref_axis',(0.,0.,-1.));
#6219=DIRECTION('center_axis',(0.,0.,1.));
#6220=DIRECTION('ref_axis',(1.,0.,0.));
#6221=DIRECTION('center_axis',(0.,-1.,0.));
#6222=DIRECTION('ref_axis',(0.,0.,-1.));
#6223=DIRECTION('center_axis',(0.,1.,0.));
#6224=DIRECTION('ref_axis',(1.,0.,0.));
#6225=DIRECTION('center_axis',(0.,-1.,0.));
#6226=DIRECTION('ref_axis',(1.,0.,0.));
#6227=DIRECTION('center_axis',(0.,-1.,0.));
#6228=DIRECTION('ref_axis',(0.,0.,-1.));
#6229=DIRECTION('center_axis',(0.,0.,1.));
#6230=DIRECTION('ref_axis',(1.,0.,0.));
#6231=DIRECTION('center_axis',(0.,-1.,0.));
#6232=DIRECTION('ref_axis',(0.,0.,-1.));
#6233=DIRECTION('center_axis',(0.,1.,0.));
#6234=DIRECTION('ref_axis',(1.,0.,0.));
#6235=DIRECTION('center_axis',(0.,1.,0.));
#6236=DIRECTION('ref_axis',(1.,0.,0.));
#6237=DIRECTION('',(0.,1.,0.));
#6238=DIRECTION('center_axis',(0.,-1.,0.));
#6239=DIRECTION('ref_axis',(1.,0.,0.));
#6240=DIRECTION('center_axis',(0.,-1.,0.));
#6241=DIRECTION('ref_axis',(1.,0.,0.));
#6242=DIRECTION('center_axis',(0.,1.,0.));
#6243=DIRECTION('ref_axis',(1.,0.,0.));
#6244=DIRECTION('center_axis',(0.,-1.,0.));
#6245=DIRECTION('ref_axis',(0.,0.,-1.));
#6246=DIRECTION('center_axis',(0.,0.,1.));
#6247=DIRECTION('ref_axis',(1.,0.,0.));
#6248=DIRECTION('center_axis',(0.,-1.,0.));
#6249=DIRECTION('ref_axis',(0.,0.,-1.));
#6250=DIRECTION('center_axis',(0.,-1.,0.));
#6251=DIRECTION('ref_axis',(-1.,0.,0.));
#6252=DIRECTION('center_axis',(0.,1.,0.));
#6253=DIRECTION('ref_axis',(1.,0.,0.));
#8705=CARTESIAN_POINT('',(0.,0.,0.));
#8706=CARTESIAN_POINT('Origin',(1.47463555300403,0.,1.23736614864659));
#8707=CARTESIAN_POINT('',(1.16188454446795,-0.07938,1.49479506783723));
#8708=CARTESIAN_POINT('',(1.67384490577674,-0.07938,0.884664467981643));
#8709=CARTESIAN_POINT('Ctrl Pts',(1.16188454446795,-0.07938,1.49479506783723));
#8710=CARTESIAN_POINT('Ctrl Pts',(1.16869700612251,-0.123392992551698,1.48949983100074));
#8711=CARTESIAN_POINT('Ctrl Pts',(1.18135446441955,-0.166529565724166,1.47962830891229));
#8712=CARTESIAN_POINT('Ctrl Pts',(1.21282145231718,-0.237213819614884,1.45388393800011));
#8713=CARTESIAN_POINT('Ctrl Pts',(1.22989120215288,-0.266247928944116,1.4395843844684));
#8714=CARTESIAN_POINT('Ctrl Pts',(1.26813946847809,-0.317173992396757,1.40600777299249));
#8715=CARTESIAN_POINT('Ctrl Pts',(1.28931069477441,-0.339063173951852,1.38671820696899));
#8716=CARTESIAN_POINT('Ctrl Pts',(1.33224261954459,-0.373566122196588,1.34549913552853));
#8717=CARTESIAN_POINT('Ctrl Pts',(1.35618281536764,-0.388075792674378,1.32151296077672));
#8718=CARTESIAN_POINT('Ctrl Pts',(1.40439359896051,-0.407069005705619,1.27016020894803));
#8719=CARTESIAN_POINT('Ctrl Pts',(1.42864614483643,-0.411552957311693,1.24277684810113));
#8720=CARTESIAN_POINT('Ctrl Pts',(1.4719780748558,-0.411552957311693,1.19113586482651));
#8721=CARTESIAN_POINT('Ctrl Pts',(1.49473401052622,-0.407069005705619,1.16249669890816));
#8722=CARTESIAN_POINT('Ctrl Pts',(1.53693488395083,-0.388075792674377,1.10610103367387));
#8723=CARTESIAN_POINT('Ctrl Pts',(1.55639948343386,-0.373566122196588,1.07835938768384));
#8724=CARTESIAN_POINT('Ctrl Pts',(1.58953729406031,-0.339063173951852,1.02892207867768));
#8725=CARTESIAN_POINT('Ctrl Pts',(1.60485746336717,-0.317173992396757,1.00472289289232));
#8726=CARTESIAN_POINT('Ctrl Pts',(1.63128222892223,-0.266247928944116,0.961225186280959));
#8727=CARTESIAN_POINT('Ctrl Pts',(1.64240040915267,-0.237213819614884,0.941931672888549));
#8728=CARTESIAN_POINT('Ctrl Pts',(1.66228948011831,-0.166529565724165,0.906472276148935));
#8729=CARTESIAN_POINT('Ctrl Pts',(1.66981308703787,-0.123392992551698,0.892292941263125));
#8730=CARTESIAN_POINT('Ctrl Pts',(1.67384490577674,-0.07938,0.884664467981643));
#8731=CARTESIAN_POINT('',(1.20622598189858,-0.07938,1.54074568637942));
#8732=CARTESIAN_POINT('Origin',(1.47463555300403,-0.07938,1.23736614864659));
#8733=CARTESIAN_POINT('',(1.72679724097776,-0.07938,0.920353018170519));
#8734=CARTESIAN_POINT('Ctrl Pts',(1.72679724097776,-0.0793800000000002,
0.920353018170518));
#8735=CARTESIAN_POINT('Ctrl Pts',(1.72470909046691,-0.10165971810728,0.92427087628551));
#8736=CARTESIAN_POINT('Ctrl Pts',(1.72169532435455,-0.123845306465941,0.929898398578877));
#8737=CARTESIAN_POINT('Ctrl Pts',(1.70911544962889,-0.192537547974292,0.952957916220029));
#8738=CARTESIAN_POINT('Ctrl Pts',(1.69580594901181,-0.236239311587943,0.976785804874841));
#8739=CARTESIAN_POINT('Ctrl Pts',(1.66527150643903,-0.303218781300911,1.02787962443771));
#8740=CARTESIAN_POINT('Ctrl Pts',(1.64438322958071,-0.3351607303803,1.06123747122987));
#8741=CARTESIAN_POINT('Ctrl Pts',(1.60730731395783,-0.3732673312795,1.11639170354769));
#8742=CARTESIAN_POINT('Ctrl Pts',(1.5873911192195,-0.387903357081022,1.1447096804553));
#8743=CARTESIAN_POINT('Ctrl Pts',(1.54427174765086,-0.40704475551587,1.20224605970712));
#8744=CARTESIAN_POINT('Ctrl Pts',(1.52104964294098,-0.411552957311693,1.23144933316771));
#8745=CARTESIAN_POINT('Ctrl Pts',(1.47686834938291,-0.411552957311693,1.284102548491));
#8746=CARTESIAN_POINT('Ctrl Pts',(1.45214121543005,-0.40704475551587,1.31204295246889));
#8747=CARTESIAN_POINT('Ctrl Pts',(1.40296654335764,-0.387903357081022,1.36449833130133));
#8748=CARTESIAN_POINT('Ctrl Pts',(1.37853719107178,-0.3732673312795,1.38902931937536));
#8749=CARTESIAN_POINT('Ctrl Pts',(1.330659040657,-0.3351607303803,1.43511940046341));
#8750=CARTESIAN_POINT('Ctrl Pts',(1.30143518572334,-0.303218781300911,1.4614828667669));
#8751=CARTESIAN_POINT('Ctrl Pts',(1.25641984639565,-0.236239311587943,1.50042577120361));
#8752=CARTESIAN_POINT('Ctrl Pts',(1.23526512743829,-0.192537547974292,1.51767074004259));
#8753=CARTESIAN_POINT('Ctrl Pts',(1.21474040800595,-0.123845306465941,1.53406374142061));
#8754=CARTESIAN_POINT('Ctrl Pts',(1.20972171541452,-0.10165971810728,1.53800893064485));
#8755=CARTESIAN_POINT('Ctrl Pts',(1.20622598189858,-0.0793800000000002,
1.54074568637942));
#8756=CARTESIAN_POINT('Origin',(1.47463555300403,-0.07938,1.23736614864659));
#8757=CARTESIAN_POINT('Origin',(0.,-0.27783,0.));
#8758=CARTESIAN_POINT('',(0.731211914226578,-0.07938,1.81499518621871));
#8759=CARTESIAN_POINT('Origin',(0.,-0.07938,0.));
#8760=CARTESIAN_POINT('',(-0.0663495263035324,-0.07938,1.95562678695688));
#8761=CARTESIAN_POINT('Ctrl Pts',(0.73121191422658,-0.0793800000000002,
1.81499518621871));
#8762=CARTESIAN_POINT('Ctrl Pts',(0.727093947478514,-0.10165971810728,1.81665420238109));
#8763=CARTESIAN_POINT('Ctrl Pts',(0.721167967091869,-0.123845306465941,
1.81902792304693));
#8764=CARTESIAN_POINT('Ctrl Pts',(0.696708851738065,-0.192537547974292,
1.82860635079188));
#8765=CARTESIAN_POINT('Ctrl Pts',(0.671196911157359,-0.236239311587943,
1.83830439039938));
#8766=CARTESIAN_POINT('Ctrl Pts',(0.614963696954177,-0.303218781300911,
1.85781736559878));
#8767=CARTESIAN_POINT('Ctrl Pts',(0.577520337936704,-0.3351607303803,1.86994423321609));
#8768=CARTESIAN_POINT('Ctrl Pts',(0.513666081644577,-0.3732673312795,1.88836288721748));
#8769=CARTESIAN_POINT('Ctrl Pts',(0.48020694664961,-0.387903357081022,1.89725383285802));
#8770=CARTESIAN_POINT('Ctrl Pts',(0.410191919979371,-0.40704475551587,1.91361265867928));
#8771=CARTESIAN_POINT('Ctrl Pts',(0.373631253366087,-0.411552957311693,
1.92105678285629));
#8772=CARTESIAN_POINT('Ctrl Pts',(0.305941584526154,-0.411552957311693,
1.932992297788));
#8773=CARTESIAN_POINT('Ctrl Pts',(0.269039755480681,-0.40704475551587,1.9385015936658));
#8774=CARTESIAN_POINT('Ctrl Pts',(0.197652103622503,-0.387903357081022,
1.94707587521355));
#8775=CARTESIAN_POINT('Ctrl Pts',(0.163169918867575,-0.3732673312795,1.95016481734985));
#8776=CARTESIAN_POINT('Ctrl Pts',(0.09686699474267,-0.3351607303803,1.95469638598893));
#8777=CARTESIAN_POINT('Ctrl Pts',(0.0575341135759475,-0.30321878130091,
1.95610724099344));
#8778=CARTESIAN_POINT('Ctrl Pts',(-0.00198165342826295,-0.236239311587942,
1.95700393417042));
#8779=CARTESIAN_POINT('Ctrl Pts',(-0.0292719606304177,-0.192537547974292,
1.95661635548909));
#8780=CARTESIAN_POINT('Ctrl Pts',(-0.0555320260694991,-0.123845306465941,
1.95598108775736));
#8781=CARTESIAN_POINT('Ctrl Pts',(-0.0619124863920986,-0.10165971810728,
1.95577732462505));
#8782=CARTESIAN_POINT('Ctrl Pts',(-0.0663495263035336,-0.0793800000000002,
1.95562678695688));
#8783=CARTESIAN_POINT('',(-0.606515593706441,-0.07938,1.86038093521056));
#8784=CARTESIAN_POINT('Origin',(0.,-0.07938,0.));
#8785=CARTESIAN_POINT('',(-1.30787935375538,-0.07938,1.45544837954646));
#8786=CARTESIAN_POINT('Ctrl Pts',(-0.60651559370644,-0.0793800000000002,
1.86038093521056));
#8787=CARTESIAN_POINT('Ctrl Pts',(-0.610736534284191,-0.10165971810728,
1.85900483732004));
#8788=CARTESIAN_POINT('Ctrl Pts',(-0.616801896862274,-0.123845306465941,
1.85701406607784));
#8789=CARTESIAN_POINT('Ctrl Pts',(-0.64169556093739,-0.192537547974292,
1.84862955113236));
#8790=CARTESIAN_POINT('Ctrl Pts',(-0.667472620950374,-0.236239311587943,
1.8396599211785));
#8791=CARTESIAN_POINT('Ctrl Pts',(-0.723092460895733,-0.303218781300911,
1.81846171405606));
#8792=CARTESIAN_POINT('Ctrl Pts',(-0.759570738251496,-0.3351607303803,1.80368330636526));
#8793=CARTESIAN_POINT('Ctrl Pts',(-0.820325219032771,-0.3732673312795,1.77674808914243));
#8794=CARTESIAN_POINT('Ctrl Pts',(-0.851671393163369,-0.387903357081022,
1.76205183123884));
#8795=CARTESIAN_POINT('Ctrl Pts',(-0.915821265825857,-0.40704475551587,
1.72957862721967));
#8796=CARTESIAN_POINT('Ctrl Pts',(-0.948613352107641,-0.411552957311693,
1.71178041367846));
#8797=CARTESIAN_POINT('Ctrl Pts',(-1.00813864789236,-0.411552957311693,
1.67741346813356));
#8798=CARTESIAN_POINT('Ctrl Pts',(-1.03994839610192,-0.40704475551587,1.65791379514105));
#8799=CARTESIAN_POINT('Ctrl Pts',(-1.10014595205605,-0.387903357081022,
1.61859497777538));
#8800=CARTESIAN_POINT('Ctrl Pts',(-1.12854637180642,-0.3732673312795,1.59879652361863));
#8801=CARTESIAN_POINT('Ctrl Pts',(-1.18225019456848,-0.3351607303803,1.55964920847973));
#8802=CARTESIAN_POINT('Ctrl Pts',(-1.21328780973407,-0.30321878130091,1.53544729744874));
#8803=CARTESIAN_POINT('Ctrl Pts',(-1.25945591558947,-0.236239311587942,
1.49787820666285));
#8804=CARTESIAN_POINT('Ctrl Pts',(-1.28011237299855,-0.192537547974292,
1.48003943283366));
#8805=CARTESIAN_POINT('Ctrl Pts',(-1.29982040797731,-0.12384530646594,1.46267314482408));
#8806=CARTESIAN_POINT('Ctrl Pts',(-1.30457714773522,-0.10165971810728,1.45841577236939));
#8807=CARTESIAN_POINT('Ctrl Pts',(-1.30787935375538,-0.0793800000000002,
1.45544837954646));
#8808=CARTESIAN_POINT('',(-1.66044771467423,-0.07938,1.03527376878636));
#8809=CARTESIAN_POINT('Origin',(0.,-0.07938,0.));
#8810=CARTESIAN_POINT('',(-1.93743789612516,-0.07938,0.274249499839291));
#8811=CARTESIAN_POINT('Ctrl Pts',(-1.66044771467423,-0.0793800000000002,
1.03527376878636));
#8812=CARTESIAN_POINT('Ctrl Pts',(-1.66279660407481,-0.10165971810728,1.03150644833954));
#8813=CARTESIAN_POINT('Ctrl Pts',(-1.66616329828505,-0.123845306465941,
1.02608268917849));
#8814=CARTESIAN_POINT('Ctrl Pts',(-1.67984348899847,-0.192537547974292,
1.00365843926907));
#8815=CARTESIAN_POINT('Ctrl Pts',(-1.69382429558355,-0.236239311587943,
0.980218129295584));
#8816=CARTESIAN_POINT('Ctrl Pts',(-1.72280562001498,-0.303218781300911,
0.928227616555729));
#8817=CARTESIAN_POINT('Ctrl Pts',(-1.74125022432338,-0.3351607303803,0.893458914759057));
#8818=CARTESIAN_POINT('Ctrl Pts',(-1.7704772328254,-0.3732673312795,0.833773113802161));
#8819=CARTESIAN_POINT('Ctrl Pts',(-1.785043222842,-0.387903357081022,0.802366194758251));
#8820=CARTESIAN_POINT('Ctrl Pts',(-1.81331150313154,-0.407044755515871,
0.736255533958675));
#8821=CARTESIAN_POINT('Ctrl Pts',(-1.82699122746714,-0.411552957311693,
0.701542964620283));
#8822=CARTESIAN_POINT('Ctrl Pts',(-1.850499602749,-0.411552957311693,0.636954234365294));
#8823=CARTESIAN_POINT('Ctrl Pts',(-1.86233313540942,-0.40704475551587,0.60156970621039));
#8824=CARTESIAN_POINT('Ctrl Pts',(-1.88317349000725,-0.387903357081022,
0.53275550155669));
#8825=CARTESIAN_POINT('Ctrl Pts',(-1.89220327271636,-0.3732673312795,0.499333567842125));
#8826=CARTESIAN_POINT('Ctrl Pts',(-1.9081793785937,-0.3351607303803,0.434824832752687));
#8827=CARTESIAN_POINT('Ctrl Pts',(-1.91639888267751,-0.30321878130091,0.396334498831876));
#8828=CARTESIAN_POINT('Ctrl Pts',(-1.92761675755301,-0.236239311587942,
0.337878619195771));
#8829=CARTESIAN_POINT('Ctrl Pts',(-1.93197397917636,-0.192537547974292,
0.310935610749289));
#8830=CARTESIAN_POINT('Ctrl Pts',(-1.93590837509782,-0.12384530646594,0.284964181626328));
#8831=CARTESIAN_POINT('Ctrl Pts',(-1.93681566289304,-0.10165971810728,0.278645271736243));
#8832=CARTESIAN_POINT('Ctrl Pts',(-1.93743789612516,-0.0793800000000002,
0.27424949983929));
#8833=CARTESIAN_POINT('',(-1.956752,-0.07938,2.39633007352518E-16));
#8834=CARTESIAN_POINT('Origin',(0.,-0.07938,0.));
#8835=CARTESIAN_POINT('',(-1.956752,-0.47628,2.39633007352518E-16));
#8836=CARTESIAN_POINT('',(-1.956752,-0.27783,2.39633007352518E-16));
#8837=CARTESIAN_POINT('Origin',(0.,-0.47628,0.));
#8838=CARTESIAN_POINT('',(-1.93743789612516,-0.07938,-0.274249499839292));
#8839=CARTESIAN_POINT('Origin',(0.,-0.07938,0.));
#8840=CARTESIAN_POINT('',(-1.66044771467423,-0.07938,-1.03527376878636));
#8841=CARTESIAN_POINT('Ctrl Pts',(-1.93743789612516,-0.0793800000000002,
-0.27424949983929));
#8842=CARTESIAN_POINT('Ctrl Pts',(-1.93681566289304,-0.10165971810728,-0.278645271736244));
#8843=CARTESIAN_POINT('Ctrl Pts',(-1.93590837509782,-0.123845306465941,
-0.284964181626328));
#8844=CARTESIAN_POINT('Ctrl Pts',(-1.93197397917636,-0.192537547974292,
-0.310935610749289));
#8845=CARTESIAN_POINT('Ctrl Pts',(-1.92761675755301,-0.236239311587942,
-0.337878619195772));
#8846=CARTESIAN_POINT('Ctrl Pts',(-1.91639888267751,-0.303218781300911,
-0.396334498831877));
#8847=CARTESIAN_POINT('Ctrl Pts',(-1.9081793785937,-0.3351607303803,-0.434824832752687));
#8848=CARTESIAN_POINT('Ctrl Pts',(-1.89220327271636,-0.3732673312795,-0.499333567842125));
#8849=CARTESIAN_POINT('Ctrl Pts',(-1.88317349000725,-0.387903357081022,
-0.53275550155669));
#8850=CARTESIAN_POINT('Ctrl Pts',(-1.86233313540942,-0.40704475551587,-0.601569706210391));
#8851=CARTESIAN_POINT('Ctrl Pts',(-1.850499602749,-0.411552957311693,-0.636954234365295));
#8852=CARTESIAN_POINT('Ctrl Pts',(-1.82699122746714,-0.411552957311693,
-0.701542964620284));
#8853=CARTESIAN_POINT('Ctrl Pts',(-1.81331150313154,-0.40704475551587,-0.736255533958675));
#8854=CARTESIAN_POINT('Ctrl Pts',(-1.785043222842,-0.387903357081022,-0.802366194758251));
#8855=CARTESIAN_POINT('Ctrl Pts',(-1.7704772328254,-0.3732673312795,-0.833773113802161));
#8856=CARTESIAN_POINT('Ctrl Pts',(-1.74125022432338,-0.3351607303803,-0.893458914759057));
#8857=CARTESIAN_POINT('Ctrl Pts',(-1.72280562001498,-0.303218781300911,
-0.92822761655573));
#8858=CARTESIAN_POINT('Ctrl Pts',(-1.69382429558355,-0.236239311587942,
-0.980218129295584));
#8859=CARTESIAN_POINT('Ctrl Pts',(-1.67984348899847,-0.192537547974292,
-1.00365843926907));
#8860=CARTESIAN_POINT('Ctrl Pts',(-1.66616329828505,-0.123845306465941,
-1.02608268917849));
#8861=CARTESIAN_POINT('Ctrl Pts',(-1.66279660407481,-0.10165971810728,-1.03150644833954));
#8862=CARTESIAN_POINT('Ctrl Pts',(-1.66044771467423,-0.0793800000000001,
-1.03527376878636));
#8863=CARTESIAN_POINT('',(-1.30787935375538,-0.07938,-1.45544837954646));
#8864=CARTESIAN_POINT('Origin',(0.,-0.07938,0.));
#8865=CARTESIAN_POINT('',(-0.60651559370644,-0.07938,-1.86038093521056));
#8866=CARTESIAN_POINT('Ctrl Pts',(-1.30787935375538,-0.0793800000000002,
-1.45544837954646));
#8867=CARTESIAN_POINT('Ctrl Pts',(-1.30457714773522,-0.10165971810728,-1.45841577236939));
#8868=CARTESIAN_POINT('Ctrl Pts',(-1.29982040797731,-0.123845306465941,
-1.46267314482408));
#8869=CARTESIAN_POINT('Ctrl Pts',(-1.28011237299855,-0.192537547974292,
-1.48003943283366));
#8870=CARTESIAN_POINT('Ctrl Pts',(-1.25945591558947,-0.236239311587942,
-1.49787820666285));
#8871=CARTESIAN_POINT('Ctrl Pts',(-1.21328780973407,-0.303218781300911,
-1.53544729744874));
#8872=CARTESIAN_POINT('Ctrl Pts',(-1.18225019456848,-0.3351607303803,-1.55964920847973));
#8873=CARTESIAN_POINT('Ctrl Pts',(-1.12854637180642,-0.3732673312795,-1.59879652361863));
#8874=CARTESIAN_POINT('Ctrl Pts',(-1.10014595205605,-0.387903357081022,
-1.61859497777538));
#8875=CARTESIAN_POINT('Ctrl Pts',(-1.03994839610192,-0.40704475551587,-1.65791379514105));
#8876=CARTESIAN_POINT('Ctrl Pts',(-1.00813864789236,-0.411552957311693,
-1.67741346813356));
#8877=CARTESIAN_POINT('Ctrl Pts',(-0.948613352107639,-0.411552957311693,
-1.71178041367846));
#8878=CARTESIAN_POINT('Ctrl Pts',(-0.915821265825855,-0.40704475551587,
-1.72957862721967));
#8879=CARTESIAN_POINT('Ctrl Pts',(-0.851671393163367,-0.387903357081022,
-1.76205183123885));
#8880=CARTESIAN_POINT('Ctrl Pts',(-0.820325219032769,-0.3732673312795,-1.77674808914243));
#8881=CARTESIAN_POINT('Ctrl Pts',(-0.759570738251494,-0.3351607303803,-1.80368330636526));
#8882=CARTESIAN_POINT('Ctrl Pts',(-0.723092460895731,-0.303218781300911,
-1.81846171405606));
#8883=CARTESIAN_POINT('Ctrl Pts',(-0.667472620950373,-0.236239311587942,
-1.8396599211785));
#8884=CARTESIAN_POINT('Ctrl Pts',(-0.641695560937389,-0.192537547974292,
-1.84862955113236));
#8885=CARTESIAN_POINT('Ctrl Pts',(-0.616801896862272,-0.123845306465941,
-1.85701406607784));
#8886=CARTESIAN_POINT('Ctrl Pts',(-0.610736534284189,-0.10165971810728,
-1.85900483732004));
#8887=CARTESIAN_POINT('Ctrl Pts',(-0.606515593706439,-0.0793800000000002,
-1.86038093521056));
#8888=CARTESIAN_POINT('',(-0.0663495263035315,-0.07938,-1.95562678695688));
#8889=CARTESIAN_POINT('Origin',(0.,-0.07938,0.));
#8890=CARTESIAN_POINT('',(0.731211914226579,-0.07938,-1.81499518621871));
#8891=CARTESIAN_POINT('Ctrl Pts',(-0.0663495263035327,-0.0793800000000002,
-1.95562678695688));
#8892=CARTESIAN_POINT('Ctrl Pts',(-0.0619124863920977,-0.10165971810728,
-1.95577732462505));
#8893=CARTESIAN_POINT('Ctrl Pts',(-0.0555320260694982,-0.123845306465941,
-1.95598108775736));
#8894=CARTESIAN_POINT('Ctrl Pts',(-0.0292719606304167,-0.192537547974292,
-1.95661635548909));
#8895=CARTESIAN_POINT('Ctrl Pts',(-0.00198165342826177,-0.236239311587943,
-1.95700393417042));
#8896=CARTESIAN_POINT('Ctrl Pts',(0.0575341135759488,-0.303218781300911,
-1.95610724099344));
#8897=CARTESIAN_POINT('Ctrl Pts',(0.0968669947426714,-0.3351607303803,-1.95469638598893));
#8898=CARTESIAN_POINT('Ctrl Pts',(0.163169918867576,-0.3732673312795,-1.95016481734985));
#8899=CARTESIAN_POINT('Ctrl Pts',(0.197652103622504,-0.387903357081022,
-1.94707587521355));
#8900=CARTESIAN_POINT('Ctrl Pts',(0.269039755480682,-0.40704475551587,-1.9385015936658));
#8901=CARTESIAN_POINT('Ctrl Pts',(0.305941584526155,-0.411552957311693,
-1.93299229778799));
#8902=CARTESIAN_POINT('Ctrl Pts',(0.373631253366089,-0.411552957311693,
-1.92105678285629));
#8903=CARTESIAN_POINT('Ctrl Pts',(0.410191919979372,-0.40704475551587,-1.91361265867928));
#8904=CARTESIAN_POINT('Ctrl Pts',(0.480206946649611,-0.387903357081022,
-1.89725383285802));
#8905=CARTESIAN_POINT('Ctrl Pts',(0.513666081644578,-0.3732673312795,-1.88836288721748));
#8906=CARTESIAN_POINT('Ctrl Pts',(0.577520337936705,-0.3351607303803,-1.86994423321609));
#8907=CARTESIAN_POINT('Ctrl Pts',(0.614963696954178,-0.30321878130091,-1.85781736559878));
#8908=CARTESIAN_POINT('Ctrl Pts',(0.67119691115736,-0.236239311587942,-1.83830439039938));
#8909=CARTESIAN_POINT('Ctrl Pts',(0.696708851738067,-0.192537547974292,
-1.82860635079188));
#8910=CARTESIAN_POINT('Ctrl Pts',(0.721167967091869,-0.123845306465941,
-1.81902792304693));
#8911=CARTESIAN_POINT('Ctrl Pts',(0.727093947478515,-0.10165971810728,-1.81665420238109));
#8912=CARTESIAN_POINT('Ctrl Pts',(0.73121191422658,-0.0793800000000002,
-1.81499518621871));
#8913=CARTESIAN_POINT('',(1.20622598189858,-0.07938,-1.54074568637942));
#8914=CARTESIAN_POINT('Origin',(0.,-0.07938,0.));
#8915=CARTESIAN_POINT('',(1.72679724097776,-0.07938,-0.920353018170518));
#8916=CARTESIAN_POINT('Ctrl Pts',(1.20622598189858,-0.0793800000000002,
-1.54074568637942));
#8917=CARTESIAN_POINT('Ctrl Pts',(1.20972171541452,-0.10165971810728,-1.53800893064485));
#8918=CARTESIAN_POINT('Ctrl Pts',(1.21474040800596,-0.123845306465941,-1.53406374142061));
#8919=CARTESIAN_POINT('Ctrl Pts',(1.23526512743829,-0.192537547974292,-1.51767074004259));
#8920=CARTESIAN_POINT('Ctrl Pts',(1.25641984639565,-0.236239311587942,-1.50042577120361));
#8921=CARTESIAN_POINT('Ctrl Pts',(1.30143518572334,-0.303218781300911,-1.4614828667669));
#8922=CARTESIAN_POINT('Ctrl Pts',(1.330659040657,-0.3351607303803,-1.43511940046341));
#8923=CARTESIAN_POINT('Ctrl Pts',(1.37853719107178,-0.3732673312795,-1.38902931937536));
#8924=CARTESIAN_POINT('Ctrl Pts',(1.40296654335764,-0.387903357081022,-1.36449833130133));
#8925=CARTESIAN_POINT('Ctrl Pts',(1.45214121543005,-0.40704475551587,-1.31204295246889));
#8926=CARTESIAN_POINT('Ctrl Pts',(1.47686834938291,-0.411552957311693,-1.284102548491));
#8927=CARTESIAN_POINT('Ctrl Pts',(1.52104964294098,-0.411552957311693,-1.23144933316771));
#8928=CARTESIAN_POINT('Ctrl Pts',(1.54427174765086,-0.407044755515871,-1.20224605970712));
#8929=CARTESIAN_POINT('Ctrl Pts',(1.5873911192195,-0.387903357081022,-1.1447096804553));
#8930=CARTESIAN_POINT('Ctrl Pts',(1.60730731395783,-0.3732673312795,-1.11639170354769));
#8931=CARTESIAN_POINT('Ctrl Pts',(1.64438322958071,-0.3351607303803,-1.06123747122987));
#8932=CARTESIAN_POINT('Ctrl Pts',(1.66527150643903,-0.303218781300911,-1.02787962443771));
#8933=CARTESIAN_POINT('Ctrl Pts',(1.69580594901181,-0.236239311587943,-0.976785804874841));
#8934=CARTESIAN_POINT('Ctrl Pts',(1.70911544962889,-0.192537547974292,-0.952957916220028));
#8935=CARTESIAN_POINT('Ctrl Pts',(1.72169532435455,-0.123845306465941,-0.929898398578876));
#8936=CARTESIAN_POINT('Ctrl Pts',(1.72470909046691,-0.10165971810728,-0.924270876285509));
#8937=CARTESIAN_POINT('Ctrl Pts',(1.72679724097776,-0.0793800000000002,
-0.920353018170518));
#8938=CARTESIAN_POINT('',(1.91439494746182,-0.07938,-0.404932555664102));
#8939=CARTESIAN_POINT('Origin',(0.,-0.07938,0.));
#8940=CARTESIAN_POINT('',(1.91439494746182,-0.07938,0.404932555664102));
#8941=CARTESIAN_POINT('Ctrl Pts',(1.91439494746182,-0.0793800000000002,
-0.404932555664103));
#8942=CARTESIAN_POINT('Ctrl Pts',(1.91531368201941,-0.10165971810728,-0.400589064950645));
#8943=CARTESIAN_POINT('Ctrl Pts',(1.91662230483958,-0.123845306465941,-0.394340921253764));
#8944=CARTESIAN_POINT('Ctrl Pts',(1.92180793393594,-0.192537547974292,-0.368590118298695));
#8945=CARTESIAN_POINT('Ctrl Pts',(1.92692853653984,-0.236239311587943,-0.341781714515643));
#8946=CARTESIAN_POINT('Ctrl Pts',(1.9363802706298,-0.303218781300911,-0.283014416607319));
#8947=CARTESIAN_POINT('Ctrl Pts',(1.94182093281998,-0.3351607303803,-0.244034097885537));
#8948=CARTESIAN_POINT('Ctrl Pts',(1.94887159083919,-0.3732673312795,-0.177951565523803));
#8949=CARTESIAN_POINT('Ctrl Pts',(1.95181734521941,-0.387903357081022,-0.143456853463462));
#8950=CARTESIAN_POINT('Ctrl Pts',(1.95576966192778,-0.40704475551587,-0.071664832078622));
#8951=CARTESIAN_POINT('Ctrl Pts',(1.956752,-0.411552957311693,-0.0343669455449008));
#8952=CARTESIAN_POINT('Ctrl Pts',(1.956752,-0.411552957311693,0.0343669455449008));
#8953=CARTESIAN_POINT('Ctrl Pts',(1.95576966192778,-0.40704475551587,0.0716648320786219));
#8954=CARTESIAN_POINT('Ctrl Pts',(1.95181734521941,-0.387903357081022,0.143456853463462));
#8955=CARTESIAN_POINT('Ctrl Pts',(1.94887159083919,-0.3732673312795,0.177951565523803));
#8956=CARTESIAN_POINT('Ctrl Pts',(1.94182093281998,-0.3351607303803,0.244034097885537));
#8957=CARTESIAN_POINT('Ctrl Pts',(1.9363802706298,-0.303218781300911,0.283014416607319));
#8958=CARTESIAN_POINT('Ctrl Pts',(1.92692853653984,-0.236239311587943,0.341781714515643));
#8959=CARTESIAN_POINT('Ctrl Pts',(1.92180793393594,-0.192537547974292,0.368590118298695));
#8960=CARTESIAN_POINT('Ctrl Pts',(1.91662230483958,-0.123845306465941,0.394340921253764));
#8961=CARTESIAN_POINT('Ctrl Pts',(1.91531368201941,-0.10165971810728,0.400589064950645));
#8962=CARTESIAN_POINT('Ctrl Pts',(1.91439494746182,-0.0793800000000002,
0.404932555664103));
#8963=CARTESIAN_POINT('Origin',(0.,-0.07938,0.));
#8964=CARTESIAN_POINT('Origin',(0.,-0.07938,0.));
#8965=CARTESIAN_POINT('',(0.71358822996475,-0.07938,1.75361906569237));
#8966=CARTESIAN_POINT('Origin',(0.,-0.07938,0.));
#8967=CARTESIAN_POINT('Origin',(0.33427274200884,-0.07938,1.8957549245485));
#8968=CARTESIAN_POINT('Origin',(0.33427274200884,0.,1.8957549245485));
#8969=CARTESIAN_POINT('',(-0.070780549790825,-0.07938,1.89192444438865));
#8970=CARTESIAN_POINT('Ctrl Pts',(-0.0707805497908251,-0.07938,1.89192444438865));
#8971=CARTESIAN_POINT('Ctrl Pts',(-0.0621581887675352,-0.123392992551698,
1.89224702357808));
#8972=CARTESIAN_POINT('Ctrl Pts',(-0.0461167210878756,-0.166529565724166,
1.89282105630055));
#8973=CARTESIAN_POINT('Ctrl Pts',(-0.00546344722567869,-0.237213819614884,
1.89332631395644));
#8974=CARTESIAN_POINT('Ctrl Pts',(0.0168043156156246,-0.266247928944116,
1.89334444412923));
#8975=CARTESIAN_POINT('Ctrl Pts',(0.0676868173249578,-0.317173992396757,
1.89220877917518));
#8976=CARTESIAN_POINT('Ctrl Pts',(0.0963040116194015,-0.339063173951852,
1.89104071625784));
#8977=CARTESIAN_POINT('Ctrl Pts',(0.155686882426711,-0.373566122196588,
1.88706118493262));
#8978=CARTESIAN_POINT('Ctrl Pts',(0.189444152338378,-0.388075792674378,
1.88407517030084));
#8979=CARTESIAN_POINT('Ctrl Pts',(0.259384667806906,-0.407069005705619,
1.87572597447038));
#8980=CARTESIAN_POINT('Ctrl Pts',(0.295564880870602,-0.411552957311693,
1.87033833905209));
#8981=CARTESIAN_POINT('Ctrl Pts',(0.361953249272518,-0.411552957311693,
1.85863227849762));
#8982=CARTESIAN_POINT('Ctrl Pts',(0.397794208344885,-0.407069005705619,
1.85132063808607));
#8983=CARTESIAN_POINT('Ctrl Pts',(0.466372387779211,-0.388075792674377,
1.83524525067264));
#8984=CARTESIAN_POINT('Ctrl Pts',(0.499115122365417,-0.373566122196588,
1.82650552029421));
#8985=CARTESIAN_POINT('Ctrl Pts',(0.55627784773835,-0.339063173951852,1.8099349185301));
#8986=CARTESIAN_POINT('Ctrl Pts',(0.583568715090836,-0.317173992396757,
1.80124488173997));
#8987=CARTESIAN_POINT('Ctrl Pts',(0.631771046764577,-0.266247928944116,
1.78490921718958));
#8988=CARTESIAN_POINT('Ctrl Pts',(0.652689698303665,-0.237213819614884,
1.77727615696148));
#8989=CARTESIAN_POINT('Ctrl Pts',(0.690718471466875,-0.166529565724165,
1.76289713151763));
#8990=CARTESIAN_POINT('Ctrl Pts',(0.705596189518013,-0.123392992551698,
1.75687121212928));
#8991=CARTESIAN_POINT('Ctrl Pts',(0.71358822996475,-0.07938,1.75361906569237));
#8992=CARTESIAN_POINT('Origin',(0.33427274200884,-0.07938,1.8957549245485));
#8993=CARTESIAN_POINT('Origin',(0.,-0.07938,0.));
#8994=CARTESIAN_POINT('',(-0.580564309297537,-0.07938,1.80203581326062));
#8995=CARTESIAN_POINT('Origin',(0.,-0.07938,0.));
#8996=CARTESIAN_POINT('Origin',(-0.962500000000001,-0.07938,1.66709890228504));
#8997=CARTESIAN_POINT('Origin',(-0.962500000000001,0.,1.66709890228504));
#8998=CARTESIAN_POINT('',(-1.27032663816428,-0.07938,1.40380134701254));
#8999=CARTESIAN_POINT('Ctrl Pts',(-1.27032663816428,-0.07938,1.40380134701254));
#9000=CARTESIAN_POINT('Ctrl Pts',(-1.26392887632193,-0.123392992551698,
1.40959080384008));
#9001=CARTESIAN_POINT('Ctrl Pts',(-1.25200938026802,-0.166529565724166,
1.42034179508297));
#9002=CARTESIAN_POINT('Ctrl Pts',(-1.22119193909219,-0.237213819614885,
1.44686026563443));
#9003=CARTESIAN_POINT('Ctrl Pts',(-1.20414549695735,-0.266247928944117,
1.46118759620237));
#9004=CARTESIAN_POINT('Ctrl Pts',(-1.16443724790971,-0.317173992396758,
1.49302426802369));
#9005=CARTESIAN_POINT('Ctrl Pts',(-1.14176438887219,-0.339063173951853,
1.51052425783311));
#9006=CARTESIAN_POINT('Ctrl Pts',(-1.09371647724559,-0.373566122196589,
1.54564633355776));
#9007=CARTESIAN_POINT('Ctrl Pts',(-1.06593753500724,-0.388075792674378,
1.56505766847808));
#9008=CARTESIAN_POINT('Ctrl Pts',(-1.00699323215303,-0.407069005705619,
1.6036187101659));
#9009=CARTESIAN_POINT('Ctrl Pts',(-0.975814475692339,-0.411552957311693,
1.62274773466534));
#9010=CARTESIAN_POINT('Ctrl Pts',(-0.917433524307661,-0.411552957311693,
1.65645399266283));
#9011=CARTESIAN_POINT('Ctrl Pts',(-0.885277924911194,-0.407069005705619,
1.67389107556648));
#9012=CARTESIAN_POINT('Ctrl Pts',(-0.822410931786043,-0.388075792674377,
1.70565781840267));
#9013=CARTESIAN_POINT('Ctrl Pts',(-0.791710751504505,-0.373566122196588,
1.72000942061118));
#9014=CARTESIAN_POINT('Ctrl Pts',(-0.737270185880016,-0.339063173951852,
1.74405909481629));
#9015=CARTESIAN_POINT('Ctrl Pts',(-0.710778320620332,-0.317173992396757,
1.75494437181449));
#9016=CARTESIAN_POINT('Ctrl Pts',(-0.663352829527299,-0.266247928944116,
1.77341438831889));
#9017=CARTESIAN_POINT('Ctrl Pts',(-0.642421776219621,-0.237213819614884,
1.78101337496783));
#9018=CARTESIAN_POINT('Ctrl Pts',(-0.604047386464641,-0.166529565724165,
1.79444282663));
#9019=CARTESIAN_POINT('Ctrl Pts',(-0.588777006905475,-0.123392992551698,
1.79938991739155));
#9020=CARTESIAN_POINT('Ctrl Pts',(-0.580564309297537,-0.0793799999999999,
1.80203581326062));
#9021=CARTESIAN_POINT('Origin',(-0.962500000000001,-0.07938,1.66709890228504));
#9022=CARTESIAN_POINT('Origin',(0.,-0.07938,0.));
#9023=CARTESIAN_POINT('',(-1.60306435598592,-0.07938,1.00725997640701));
#9024=CARTESIAN_POINT('Origin',(0.,-0.07938,0.));
#9025=CARTESIAN_POINT('Origin',(-1.80890829501287,-0.07938,0.658388775901912));
#9026=CARTESIAN_POINT('Origin',(-1.80890829501287,0.,0.658388775901912));
#9027=CARTESIAN_POINT('',(-1.8754727744327,-0.07938,0.258823997855139));
#9028=CARTESIAN_POINT('Ctrl Pts',(-1.8754727744327,-0.07938,0.258823997855138));
#9029=CARTESIAN_POINT('Ctrl Pts',(-1.87429319564052,-0.123392992551698,
0.267371381128541));
#9030=CARTESIAN_POINT('Ctrl Pts',(-1.87207293588642,-0.166529565724165,
0.283268822605344));
#9031=CARTESIAN_POINT('Ctrl Pts',(-1.86551115062085,-0.237213819614884,
0.323392218961362));
#9032=CARTESIAN_POINT('Ctrl Pts',(-1.86166224891746,-0.266247928944116,
0.34532483272118));
#9033=CARTESIAN_POINT('Ctrl Pts',(-1.85170818356893,-0.317173992396757,
0.395237108747477));
#9034=CARTESIAN_POINT('Ctrl Pts',(-1.84558854251276,-0.339063173951852,
0.423216711561106));
#9035=CARTESIAN_POINT('Ctrl Pts',(-1.83135774191,-0.373566122196588,0.481006384765672));
#9036=CARTESIAN_POINT('Ctrl Pts',(-1.82255520314685,-0.388075792674377,
0.513732289895913));
#9037=CARTESIAN_POINT('Ctrl Pts',(-1.8021878073054,-0.407069005705619,0.581160429138046));
#9038=CARTESIAN_POINT('Ctrl Pts',(-1.79059939410895,-0.411552957311693,
0.615855430396488));
#9039=CARTESIAN_POINT('Ctrl Pts',(-1.76754295572641,-0.411552957311693,
0.679202474225583));
#9040=CARTESIAN_POINT('Ctrl Pts',(-1.75411867833313,-0.407069005705619,
0.713229275562222));
#9041=CARTESIAN_POINT('Ctrl Pts',(-1.72637903628921,-0.388075792674378,
0.777974136626975));
#9042=CARTESIAN_POINT('Ctrl Pts',(-1.71208636586057,-0.373566122196588,
0.808701797248777));
#9043=CARTESIAN_POINT('Ctrl Pts',(-1.68584130567972,-0.339063173951852,
0.862118637580169));
#9044=CARTESIAN_POINT('Ctrl Pts',(-1.67254428069212,-0.317173992396757,
0.88748588628286));
#9045=CARTESIAN_POINT('Ctrl Pts',(-1.64808654453785,-0.266247928944116,
0.932119257848273));
#9046=CARTESIAN_POINT('Ctrl Pts',(-1.63693696192699,-0.237213819614884,
0.951394641067894));
#9047=CARTESIAN_POINT('Ctrl Pts',(-1.61617275903043,-0.166529565724165,
0.986348780151617));
#9048=CARTESIAN_POINT('Ctrl Pts',(-1.60765489827034,-0.123392992551698,
0.999954082314951));
#9049=CARTESIAN_POINT('Ctrl Pts',(-1.60306435598592,-0.07938,1.00725997640701));
#9050=CARTESIAN_POINT('Origin',(-1.80890829501287,-0.07938,0.658388775901912));
#9051=CARTESIAN_POINT('Origin',(0.,-0.07938,0.));
#9052=CARTESIAN_POINT('',(-1.893248,-0.0793799999999999,2.31856010319213E-16));
#9053=CARTESIAN_POINT('Origin',(0.,-0.07938,0.));
#9054=CARTESIAN_POINT('',(-1.8754727744327,-0.07938,-0.258823997855139));
#9055=CARTESIAN_POINT('Origin',(0.,-0.07938,0.));
#9056=CARTESIAN_POINT('Origin',(-1.80890829501287,-0.07938,-0.658388775901913));
#9057=CARTESIAN_POINT('Origin',(-1.80890829501287,0.,-0.658388775901913));
#9058=CARTESIAN_POINT('',(-1.60306435598592,-0.07938,-1.00725997640701));
#9059=CARTESIAN_POINT('Ctrl Pts',(-1.60306435598592,-0.07938,-1.00725997640701));
#9060=CARTESIAN_POINT('Ctrl Pts',(-1.60765489827034,-0.123392992551698,
-0.999954082314952));
#9061=CARTESIAN_POINT('Ctrl Pts',(-1.61617275903043,-0.166529565724166,
-0.986348780151617));
#9062=CARTESIAN_POINT('Ctrl Pts',(-1.63693696192699,-0.237213819614884,
-0.951394641067894));
#9063=CARTESIAN_POINT('Ctrl Pts',(-1.64808654453785,-0.266247928944116,
-0.932119257848273));
#9064=CARTESIAN_POINT('Ctrl Pts',(-1.67254428069212,-0.317173992396757,
-0.88748588628286));
#9065=CARTESIAN_POINT('Ctrl Pts',(-1.68584130567972,-0.339063173951852,
-0.862118637580169));
#9066=CARTESIAN_POINT('Ctrl Pts',(-1.71208636586057,-0.373566122196588,
-0.808701797248777));
#9067=CARTESIAN_POINT('Ctrl Pts',(-1.72637903628921,-0.388075792674377,
-0.777974136626975));
#9068=CARTESIAN_POINT('Ctrl Pts',(-1.75411867833313,-0.407069005705619,
-0.713229275562223));
#9069=CARTESIAN_POINT('Ctrl Pts',(-1.76754295572641,-0.411552957311693,
-0.679202474225584));
#9070=CARTESIAN_POINT('Ctrl Pts',(-1.79059939410895,-0.411552957311693,
-0.615855430396488));
#9071=CARTESIAN_POINT('Ctrl Pts',(-1.8021878073054,-0.407069005705619,-0.581160429138047));
#9072=CARTESIAN_POINT('Ctrl Pts',(-1.82255520314685,-0.388075792674378,
-0.513732289895914));
#9073=CARTESIAN_POINT('Ctrl Pts',(-1.83135774191,-0.373566122196588,-0.481006384765673));
#9074=CARTESIAN_POINT('Ctrl Pts',(-1.84558854251276,-0.339063173951852,
-0.423216711561107));
#9075=CARTESIAN_POINT('Ctrl Pts',(-1.85170818356893,-0.317173992396757,
-0.395237108747477));
#9076=CARTESIAN_POINT('Ctrl Pts',(-1.86166224891746,-0.266247928944116,
-0.34532483272118));
#9077=CARTESIAN_POINT('Ctrl Pts',(-1.86551115062085,-0.237213819614884,
-0.323392218961362));
#9078=CARTESIAN_POINT('Ctrl Pts',(-1.87207293588642,-0.166529565724166,
-0.283268822605344));
#9079=CARTESIAN_POINT('Ctrl Pts',(-1.87429319564052,-0.123392992551698,
-0.267371381128542));
#9080=CARTESIAN_POINT('Ctrl Pts',(-1.8754727744327,-0.07938,-0.258823997855139));
#9081=CARTESIAN_POINT('Origin',(-1.80890829501287,-0.07938,-0.658388775901913));
#9082=CARTESIAN_POINT('Origin',(0.,-0.07938,0.));
#9083=CARTESIAN_POINT('',(-1.27032663816428,-0.07938,-1.40380134701254));
#9084=CARTESIAN_POINT('Origin',(0.,-0.07938,0.));
#9085=CARTESIAN_POINT('Origin',(-0.9625,-0.07938,-1.66709890228504));
#9086=CARTESIAN_POINT('Origin',(-0.9625,0.,-1.66709890228504));
#9087=CARTESIAN_POINT('',(-0.580564309297535,-0.07938,-1.80203581326062));
#9088=CARTESIAN_POINT('Ctrl Pts',(-0.580564309297535,-0.07938,-1.80203581326062));
#9089=CARTESIAN_POINT('Ctrl Pts',(-0.588777006905474,-0.123392992551698,
-1.79938991739155));
#9090=CARTESIAN_POINT('Ctrl Pts',(-0.60404738646464,-0.166529565724165,
-1.79444282663));
#9091=CARTESIAN_POINT('Ctrl Pts',(-0.642421776219619,-0.237213819614884,
-1.78101337496783));
#9092=CARTESIAN_POINT('Ctrl Pts',(-0.663352829527298,-0.266247928944116,
-1.77341438831889));
#9093=CARTESIAN_POINT('Ctrl Pts',(-0.71077832062033,-0.317173992396757,
-1.75494437181449));
#9094=CARTESIAN_POINT('Ctrl Pts',(-0.737270185880015,-0.339063173951852,
-1.74405909481629));
#9095=CARTESIAN_POINT('Ctrl Pts',(-0.791710751504504,-0.373566122196588,
-1.72000942061118));
#9096=CARTESIAN_POINT('Ctrl Pts',(-0.822410931786042,-0.388075792674378,
-1.70565781840267));
#9097=CARTESIAN_POINT('Ctrl Pts',(-0.885277924911194,-0.407069005705619,
-1.67389107556648));
#9098=CARTESIAN_POINT('Ctrl Pts',(-0.917433524307661,-0.411552957311693,
-1.65645399266283));
#9099=CARTESIAN_POINT('Ctrl Pts',(-0.975814475692338,-0.411552957311693,
-1.62274773466534));
#9100=CARTESIAN_POINT('Ctrl Pts',(-1.00699323215303,-0.407069005705619,
-1.60361871016591));
#9101=CARTESIAN_POINT('Ctrl Pts',(-1.06593753500724,-0.388075792674378,
-1.56505766847808));
#9102=CARTESIAN_POINT('Ctrl Pts',(-1.09371647724559,-0.373566122196588,
-1.54564633355776));
#9103=CARTESIAN_POINT('Ctrl Pts',(-1.14176438887219,-0.339063173951852,
-1.51052425783311));
#9104=CARTESIAN_POINT('Ctrl Pts',(-1.1644372479097,-0.317173992396757,-1.49302426802369));
#9105=CARTESIAN_POINT('Ctrl Pts',(-1.20414549695735,-0.266247928944116,
-1.46118759620237));
#9106=CARTESIAN_POINT('Ctrl Pts',(-1.22119193909219,-0.237213819614884,
-1.44686026563443));
#9107=CARTESIAN_POINT('Ctrl Pts',(-1.25200938026802,-0.166529565724166,
-1.42034179508298));
#9108=CARTESIAN_POINT('Ctrl Pts',(-1.26392887632193,-0.123392992551698,
-1.40959080384008));
#9109=CARTESIAN_POINT('Ctrl Pts',(-1.27032663816428,-0.07938,-1.40380134701254));
#9110=CARTESIAN_POINT('Origin',(-0.9625,-0.07938,-1.66709890228504));
#9111=CARTESIAN_POINT('Origin',(0.,-0.07938,0.));
#9112=CARTESIAN_POINT('',(-0.0707805497908242,-0.07938,-1.89192444438865));
#9113=CARTESIAN_POINT('Origin',(0.,-0.07938,0.));
#9114=CARTESIAN_POINT('Origin',(0.334272742008841,-0.07938,-1.8957549245485));
#9115=CARTESIAN_POINT('Origin',(0.334272742008841,0.,-1.8957549245485));
#9116=CARTESIAN_POINT('',(0.71358822996475,-0.07938,-1.75361906569237));
#9117=CARTESIAN_POINT('Ctrl Pts',(0.71358822996475,-0.07938,-1.75361906569237));
#9118=CARTESIAN_POINT('Ctrl Pts',(0.705596189518014,-0.123392992551698,
-1.75687121212928));
#9119=CARTESIAN_POINT('Ctrl Pts',(0.690718471466876,-0.166529565724166,
-1.76289713151763));
#9120=CARTESIAN_POINT('Ctrl Pts',(0.652689698303666,-0.237213819614884,
-1.77727615696148));
#9121=CARTESIAN_POINT('Ctrl Pts',(0.631771046764578,-0.266247928944116,
-1.78490921718958));
#9122=CARTESIAN_POINT('Ctrl Pts',(0.583568715090837,-0.317173992396757,
-1.80124488173997));
#9123=CARTESIAN_POINT('Ctrl Pts',(0.556277847738351,-0.339063173951852,
-1.8099349185301));
#9124=CARTESIAN_POINT('Ctrl Pts',(0.499115122365417,-0.373566122196588,
-1.8265055202942));
#9125=CARTESIAN_POINT('Ctrl Pts',(0.466372387779211,-0.388075792674378,
-1.83524525067263));
#9126=CARTESIAN_POINT('Ctrl Pts',(0.397794208344886,-0.407069005705619,
-1.85132063808607));
#9127=CARTESIAN_POINT('Ctrl Pts',(0.361953249272519,-0.411552957311693,
-1.85863227849762));
#9128=CARTESIAN_POINT('Ctrl Pts',(0.295564880870602,-0.411552957311693,
-1.87033833905209));
#9129=CARTESIAN_POINT('Ctrl Pts',(0.259384667806906,-0.407069005705619,
-1.87572597447038));
#9130=CARTESIAN_POINT('Ctrl Pts',(0.189444152338379,-0.388075792674377,
-1.88407517030084));
#9131=CARTESIAN_POINT('Ctrl Pts',(0.155686882426711,-0.373566122196588,
-1.88706118493262));
#9132=CARTESIAN_POINT('Ctrl Pts',(0.096304011619402,-0.339063173951852,
-1.89104071625784));
#9133=CARTESIAN_POINT('Ctrl Pts',(0.0676868173249583,-0.317173992396757,
-1.89220877917518));
#9134=CARTESIAN_POINT('Ctrl Pts',(0.0168043156156251,-0.266247928944116,
-1.89334444412923));
#9135=CARTESIAN_POINT('Ctrl Pts',(-0.00546344722567807,-0.237213819614884,
-1.89332631395644));
#9136=CARTESIAN_POINT('Ctrl Pts',(-0.0461167210878748,-0.166529565724165,
-1.89282105630055));
#9137=CARTESIAN_POINT('Ctrl Pts',(-0.0621581887675344,-0.123392992551698,
-1.89224702357808));
#9138=CARTESIAN_POINT('Ctrl Pts',(-0.0707805497908242,-0.07938,-1.89192444438865));
#9139=CARTESIAN_POINT('Origin',(0.334272742008841,-0.07938,-1.8957549245485));
#9140=CARTESIAN_POINT('Origin',(0.,-0.07938,0.));
#9141=CARTESIAN_POINT('',(1.16188454446795,-0.07938,-1.49479506783723));
#9142=CARTESIAN_POINT('Origin',(0.,-0.07938,0.));
#9143=CARTESIAN_POINT('Origin',(1.47463555300403,-0.07938,-1.23736614864659));
#9144=CARTESIAN_POINT('Origin',(1.47463555300403,0.,-1.23736614864659));
#9145=CARTESIAN_POINT('',(1.67384490577674,-0.07938,-0.884664467981643));
#9146=CARTESIAN_POINT('Ctrl Pts',(1.67384490577674,-0.07938,-0.884664467981643));
#9147=CARTESIAN_POINT('Ctrl Pts',(1.66981308703787,-0.123392992551698,-0.892292941263125));
#9148=CARTESIAN_POINT('Ctrl Pts',(1.66228948011831,-0.166529565724165,-0.906472276148934));
#9149=CARTESIAN_POINT('Ctrl Pts',(1.64240040915267,-0.237213819614884,-0.941931672888549));
#9150=CARTESIAN_POINT('Ctrl Pts',(1.63128222892223,-0.266247928944116,-0.961225186280958));
#9151=CARTESIAN_POINT('Ctrl Pts',(1.60485746336717,-0.317173992396757,-1.00472289289232));
#9152=CARTESIAN_POINT('Ctrl Pts',(1.58953729406031,-0.339063173951852,-1.02892207867768));
#9153=CARTESIAN_POINT('Ctrl Pts',(1.55639948343386,-0.373566122196588,-1.07835938768384));
#9154=CARTESIAN_POINT('Ctrl Pts',(1.53693488395083,-0.388075792674377,-1.10610103367386));
#9155=CARTESIAN_POINT('Ctrl Pts',(1.49473401052622,-0.407069005705619,-1.16249669890816));
#9156=CARTESIAN_POINT('Ctrl Pts',(1.4719780748558,-0.411552957311693,-1.19113586482651));
#9157=CARTESIAN_POINT('Ctrl Pts',(1.42864614483643,-0.411552957311693,-1.24277684810113));
#9158=CARTESIAN_POINT('Ctrl Pts',(1.40439359896051,-0.407069005705619,-1.27016020894803));
#9159=CARTESIAN_POINT('Ctrl Pts',(1.35618281536764,-0.388075792674378,-1.32151296077672));
#9160=CARTESIAN_POINT('Ctrl Pts',(1.33224261954459,-0.373566122196588,-1.34549913552853));
#9161=CARTESIAN_POINT('Ctrl Pts',(1.28931069477441,-0.339063173951852,-1.38671820696899));
#9162=CARTESIAN_POINT('Ctrl Pts',(1.26813946847809,-0.317173992396757,-1.40600777299249));
#9163=CARTESIAN_POINT('Ctrl Pts',(1.22989120215289,-0.266247928944116,-1.4395843844684));
#9164=CARTESIAN_POINT('Ctrl Pts',(1.21282145231718,-0.237213819614884,-1.45388393800011));
#9165=CARTESIAN_POINT('Ctrl Pts',(1.18135446441955,-0.166529565724166,-1.47962830891229));
#9166=CARTESIAN_POINT('Ctrl Pts',(1.16869700612251,-0.123392992551698,-1.48949983100074));
#9167=CARTESIAN_POINT('Ctrl Pts',(1.16188454446795,-0.0793799999999999,
-1.49479506783723));
#9168=CARTESIAN_POINT('Origin',(1.47463555300403,-0.07938,-1.23736614864659));
#9169=CARTESIAN_POINT('Origin',(0.,-0.27783,0.));
#9170=CARTESIAN_POINT('',(-1.893248,-0.47628,2.31856010319213E-16));
#9171=CARTESIAN_POINT('Origin',(0.,-0.47628,0.));
#9172=CARTESIAN_POINT('',(-1.893248,-0.27783,2.31856010319213E-16));
#9173=CARTESIAN_POINT('',(1.85089094746182,-0.07938,0.39823446624808));
#9174=CARTESIAN_POINT('Origin',(0.,-0.07938,0.));
#9175=CARTESIAN_POINT('',(1.85089094746182,-0.07938,-0.39823446624808));
#9176=CARTESIAN_POINT('Ctrl Pts',(1.85089094746182,-0.07938,0.39823446624808));
#9177=CARTESIAN_POINT('Ctrl Pts',(1.8527058832274,-0.123392992551698,0.38979911355147));
#9178=CARTESIAN_POINT('Ctrl Pts',(1.85605676673266,-0.166529565724166,0.374101031547026));
#9179=CARTESIAN_POINT('Ctrl Pts',(1.86361371531181,-0.237213819614884,0.334153109333404));
#9180=CARTESIAN_POINT('Ctrl Pts',(1.86749832648465,-0.266247928944116,0.312226792116516));
#9181=CARTESIAN_POINT('Ctrl Pts',(1.87521556853004,-0.317173992396757,0.261920103790797));
#9182=CARTESIAN_POINT('Ctrl Pts',(1.87903457475221,-0.339063173951852,0.233534836983177));
#9183=CARTESIAN_POINT('Ctrl Pts',(1.88542722875009,-0.373566122196588,0.174363087053423));
#9184=CARTESIAN_POINT('Ctrl Pts',(1.88834846679328,-0.388075792674378,0.140600149924591));
#9185=CARTESIAN_POINT('Ctrl Pts',(1.89227115706422,-0.407069005705619,0.0702723654005715));
#9186=CARTESIAN_POINT('Ctrl Pts',(1.893248,-0.411552957311693,0.0337062579974903));
#9187=CARTESIAN_POINT('Ctrl Pts',(1.893248,-0.411552957311693,-0.0337062579974903));
#9188=CARTESIAN_POINT('Ctrl Pts',(1.89227115706422,-0.407069005705619,-0.0702723654005715));
#9189=CARTESIAN_POINT('Ctrl Pts',(1.88834846679328,-0.388075792674378,-0.140600149924591));
#9190=CARTESIAN_POINT('Ctrl Pts',(1.88542722875009,-0.373566122196588,-0.174363087053422));
#9191=CARTESIAN_POINT('Ctrl Pts',(1.87903457475221,-0.339063173951852,-0.233534836983177));
#9192=CARTESIAN_POINT('Ctrl Pts',(1.87521556853004,-0.317173992396757,-0.261920103790797));
#9193=CARTESIAN_POINT('Ctrl Pts',(1.86749832648465,-0.266247928944116,-0.312226792116516));
#9194=CARTESIAN_POINT('Ctrl Pts',(1.86361371531181,-0.237213819614884,-0.334153109333404));
#9195=CARTESIAN_POINT('Ctrl Pts',(1.85605676673266,-0.166529565724166,-0.374101031547026));
#9196=CARTESIAN_POINT('Ctrl Pts',(1.8527058832274,-0.123392992551698,-0.38979911355147));
#9197=CARTESIAN_POINT('Ctrl Pts',(1.85089094746182,-0.07938,-0.39823446624808));
#9198=CARTESIAN_POINT('Origin',(0.,-0.07938,0.));
#9199=CARTESIAN_POINT('Origin',(0.,-0.07938,0.));
#9200=CARTESIAN_POINT('Origin',(1.925,-0.07938,0.));
#9201=CARTESIAN_POINT('Origin',(1.925,0.,0.));
#9202=CARTESIAN_POINT('Origin',(1.925,-0.07938,0.));
#9203=CARTESIAN_POINT('Origin',(0.,-0.47628,0.));
#9204=CARTESIAN_POINT('Origin',(0.,-0.07938,0.));
#9974=UNCERTAINTY_MEASURE_WITH_UNIT(LENGTH_MEASURE(0.001),#10021,
'DISTANCE_ACCURACY_VALUE',
'Maximum model space distance between geometric entities at asserted c
onnectivities');
#9987=UNCERTAINTY_MEASURE_WITH_UNIT(LENGTH_MEASURE(0.001),#10021,
'DISTANCE_ACCURACY_VALUE',
'Maximum model space distance between geometric entities at asserted c
onnectivities');
#10007=(
GEOMETRIC_REPRESENTATION_CONTEXT(3)
GLOBAL_UNCERTAINTY_ASSIGNED_CONTEXT((#9974))
GLOBAL_UNIT_ASSIGNED_CONTEXT((#10021,#10023,#10024))
REPRESENTATION_CONTEXT('','3D')
);
#10020=(
GEOMETRIC_REPRESENTATION_CONTEXT(3)
GLOBAL_UNCERTAINTY_ASSIGNED_CONTEXT((#9987))
GLOBAL_UNIT_ASSIGNED_CONTEXT((#10021,#10023,#10024))
REPRESENTATION_CONTEXT('','3D')
);
#10021=(
LENGTH_UNIT()
NAMED_UNIT(*)
SI_UNIT(.CENTI.,.METRE.)
);
#10023=(
NAMED_UNIT(*)
PLANE_ANGLE_UNIT()
SI_UNIT($,.RADIAN.)
);
#10024=(
NAMED_UNIT(*)
SI_UNIT($,.STERADIAN.)
SOLID_ANGLE_UNIT()
);
#10044=SHAPE_DEFINITION_REPRESENTATION(#10076,#10154);
#10076=PRODUCT_DEFINITION_SHAPE('',$,#10187);
#10154=SHAPE_REPRESENTATION('',(#5144),#10007);
#10167=PRODUCT_DEFINITION_CONTEXT('part definition',#10265,'design');
#10187=PRODUCT_DEFINITION('Cage','Cage',#10219,#10167);
#10219=PRODUCT_DEFINITION_FORMATION('',$,#10286);
#10265=APPLICATION_CONTEXT(
'Core Data for Automotive Mechanical Design Process');
#10266=PRODUCT_CONTEXT('part definition',#10265,'mechanical');
#10286=PRODUCT('Cage','Cage','Cage',(#10266));
#10362=COLOUR_RGB('Grey',0.48,0.52,0.57);
#10363=FILL_AREA_STYLE_COLOUR('',#10362);
#10364=FILL_AREA_STYLE('',(#10363));
#10365=SURFACE_STYLE_FILL_AREA(#10364);
#10366=SURFACE_SIDE_STYLE('',(#10365));
#10367=SURFACE_STYLE_USAGE(.BOTH.,#10366);
#10368=PRESENTATION_STYLE_ASSIGNMENT((#10367));
ENDSEC;
END-ISO-10303-21;
